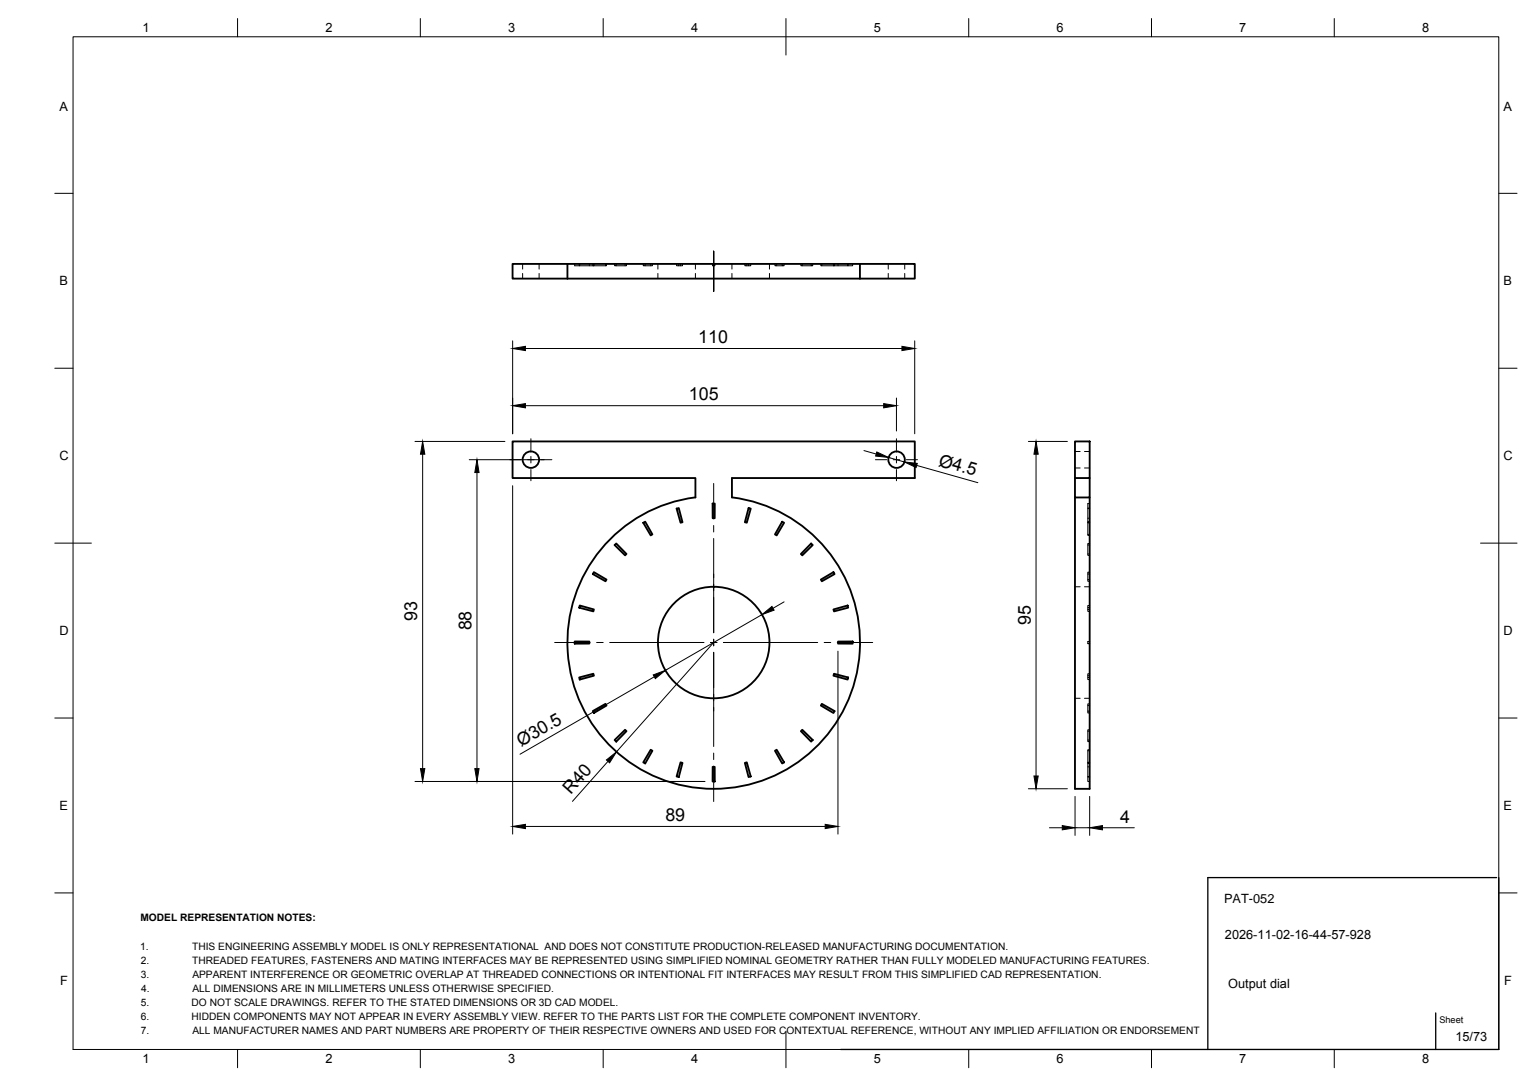
ISO-10303-21;
HEADER;
/* Generated by software containing ST-Developer
 * from STEP Tools, Inc. (www.steptools.com) 
 */

FILE_DESCRIPTION(
/* description */ ('Hand-crank gear train demonstrator'),
/* implementation_level */ '2;1');

FILE_NAME(
/* name */ 'Output dial.step',
/* time_stamp */ '2026-10-28T03:22:13-07:00',
/* author */ (''),
/* organization */ (''),
/* preprocessor_version */ 'ST-DEVELOPER v20.2',
/* originating_system */ 'Autodesk Translation Framework v15.17.0.0',
/* authorisation */ '');

FILE_SCHEMA (('AUTOMOTIVE_DESIGN { 1 0 10303 214 3 1 1 }'));
ENDSEC;

DATA;
#10=MECHANICAL_DESIGN_GEOMETRIC_PRESENTATION_REPRESENTATION('',(#1226),#62758);
#1083=SHAPE_REPRESENTATION_RELATIONSHIP('SRR','None',#63057,#1147);
#1147=ADVANCED_BREP_SHAPE_REPRESENTATION('',(#1303),#62711);
#1226=STYLED_ITEM('',(#63476),#1303);
#1303=MANIFOLD_SOLID_BREP('Body1',#16408);
#1506=FACE_BOUND('',#3606,.T.);
#1507=FACE_BOUND('',#3607,.T.);
#1508=FACE_BOUND('',#3608,.T.);
#1509=FACE_BOUND('',#3611,.T.);
#1510=FACE_BOUND('',#3612,.T.);
#1511=FACE_BOUND('',#3613,.T.);
#1512=FACE_BOUND('',#3614,.T.);
#1513=FACE_BOUND('',#3615,.T.);
#1514=FACE_BOUND('',#3616,.T.);
#1515=FACE_BOUND('',#3617,.T.);
#1516=FACE_BOUND('',#3618,.T.);
#1517=FACE_BOUND('',#3619,.T.);
#1518=FACE_BOUND('',#3620,.T.);
#1519=FACE_BOUND('',#3621,.T.);
#1520=FACE_BOUND('',#3622,.T.);
#1521=FACE_BOUND('',#3623,.T.);
#1522=FACE_BOUND('',#3624,.T.);
#1523=FACE_BOUND('',#3625,.T.);
#1524=FACE_BOUND('',#3626,.T.);
#1525=FACE_BOUND('',#3627,.T.);
#1526=FACE_BOUND('',#3628,.T.);
#1527=FACE_BOUND('',#3629,.T.);
#1528=FACE_BOUND('',#3630,.T.);
#1529=FACE_BOUND('',#3631,.T.);
#1530=FACE_BOUND('',#3632,.T.);
#1531=FACE_BOUND('',#3633,.T.);
#1532=FACE_BOUND('',#3634,.T.);
#1533=FACE_BOUND('',#3635,.T.);
#1534=FACE_BOUND('',#3636,.T.);
#1535=FACE_BOUND('',#3637,.T.);
#1726=PLANE('',#17771);
#1727=PLANE('',#17772);
#1728=PLANE('',#17773);
#1729=PLANE('',#17774);
#1730=PLANE('',#17775);
#1731=PLANE('',#17776);
#1732=PLANE('',#17777);
#1733=PLANE('',#17778);
#1734=PLANE('',#17779);
#1735=PLANE('',#17780);
#1736=PLANE('',#17781);
#1737=PLANE('',#17782);
#1738=PLANE('',#17783);
#1739=PLANE('',#17784);
#1740=PLANE('',#17785);
#1741=PLANE('',#17786);
#1742=PLANE('',#17787);
#1743=PLANE('',#17788);
#1744=PLANE('',#17789);
#1745=PLANE('',#17790);
#1746=PLANE('',#17791);
#1747=PLANE('',#17792);
#1748=PLANE('',#17793);
#1749=PLANE('',#17794);
#1750=PLANE('',#17795);
#1751=PLANE('',#17796);
#1752=PLANE('',#17797);
#1753=PLANE('',#17798);
#1754=PLANE('',#17799);
#1755=PLANE('',#17800);
#1756=PLANE('',#17801);
#1757=PLANE('',#17802);
#1758=PLANE('',#17803);
#1759=PLANE('',#17804);
#1760=PLANE('',#17805);
#1761=PLANE('',#17806);
#1762=PLANE('',#17807);
#1763=PLANE('',#17808);
#1764=PLANE('',#17809);
#1765=PLANE('',#17810);
#1766=PLANE('',#17811);
#1767=PLANE('',#17812);
#1768=PLANE('',#17813);
#1769=PLANE('',#17814);
#1770=PLANE('',#17815);
#1771=PLANE('',#17816);
#1772=PLANE('',#17817);
#1773=PLANE('',#17818);
#1774=PLANE('',#17819);
#1775=PLANE('',#17820);
#1776=PLANE('',#17821);
#1777=PLANE('',#17822);
#1778=PLANE('',#17823);
#1779=PLANE('',#17824);
#1780=PLANE('',#17825);
#1781=PLANE('',#17826);
#1782=PLANE('',#17827);
#1783=PLANE('',#17828);
#1784=PLANE('',#17829);
#1785=PLANE('',#17830);
#1786=PLANE('',#17831);
#1787=PLANE('',#17832);
#1788=PLANE('',#17833);
#1789=PLANE('',#17834);
#1790=PLANE('',#17835);
#1791=PLANE('',#17836);
#1792=PLANE('',#17837);
#1793=PLANE('',#17838);
#1794=PLANE('',#17839);
#1795=PLANE('',#17840);
#1796=PLANE('',#17841);
#1797=PLANE('',#17842);
#1798=PLANE('',#17843);
#1799=PLANE('',#17844);
#1800=PLANE('',#17845);
#1801=PLANE('',#17846);
#1802=PLANE('',#17847);
#1803=PLANE('',#17848);
#1804=PLANE('',#17849);
#1805=PLANE('',#17850);
#1806=PLANE('',#17851);
#1807=PLANE('',#17852);
#1808=PLANE('',#17853);
#1809=PLANE('',#17854);
#1810=PLANE('',#17855);
#1811=PLANE('',#17856);
#1812=PLANE('',#17857);
#1813=PLANE('',#17858);
#1814=PLANE('',#17859);
#1815=PLANE('',#17860);
#1816=PLANE('',#17861);
#1817=PLANE('',#17862);
#1818=PLANE('',#17863);
#1819=PLANE('',#17864);
#1820=PLANE('',#17865);
#1821=PLANE('',#17866);
#1822=PLANE('',#17867);
#1823=PLANE('',#17868);
#1824=PLANE('',#17869);
#1825=PLANE('',#17870);
#1826=PLANE('',#17871);
#1827=PLANE('',#17872);
#1828=PLANE('',#17873);
#1829=PLANE('',#17874);
#1830=PLANE('',#17875);
#1831=PLANE('',#17876);
#1832=PLANE('',#17877);
#1833=PLANE('',#17878);
#1834=PLANE('',#17879);
#1835=PLANE('',#17880);
#1836=PLANE('',#17881);
#1837=PLANE('',#17882);
#1838=PLANE('',#17883);
#1839=PLANE('',#17884);
#1840=PLANE('',#17885);
#1841=PLANE('',#17886);
#1842=PLANE('',#17887);
#1843=PLANE('',#17888);
#1844=PLANE('',#17889);
#1845=PLANE('',#17890);
#1846=PLANE('',#17900);
#1847=PLANE('',#17901);
#1848=PLANE('',#17902);
#1849=PLANE('',#17903);
#1850=PLANE('',#17904);
#1851=PLANE('',#17905);
#1852=PLANE('',#17906);
#1853=PLANE('',#17908);
#1854=PLANE('',#17909);
#2376=FACE_OUTER_BOUND('',#3476,.T.);
#2377=FACE_OUTER_BOUND('',#3477,.T.);
#2378=FACE_OUTER_BOUND('',#3478,.T.);
#2379=FACE_OUTER_BOUND('',#3479,.T.);
#2380=FACE_OUTER_BOUND('',#3480,.T.);
#2381=FACE_OUTER_BOUND('',#3481,.T.);
#2382=FACE_OUTER_BOUND('',#3482,.T.);
#2383=FACE_OUTER_BOUND('',#3483,.T.);
#2384=FACE_OUTER_BOUND('',#3484,.T.);
#2385=FACE_OUTER_BOUND('',#3485,.T.);
#2386=FACE_OUTER_BOUND('',#3486,.T.);
#2387=FACE_OUTER_BOUND('',#3487,.T.);
#2388=FACE_OUTER_BOUND('',#3488,.T.);
#2389=FACE_OUTER_BOUND('',#3489,.T.);
#2390=FACE_OUTER_BOUND('',#3490,.T.);
#2391=FACE_OUTER_BOUND('',#3491,.T.);
#2392=FACE_OUTER_BOUND('',#3492,.T.);
#2393=FACE_OUTER_BOUND('',#3493,.T.);
#2394=FACE_OUTER_BOUND('',#3494,.T.);
#2395=FACE_OUTER_BOUND('',#3495,.T.);
#2396=FACE_OUTER_BOUND('',#3496,.T.);
#2397=FACE_OUTER_BOUND('',#3497,.T.);
#2398=FACE_OUTER_BOUND('',#3498,.T.);
#2399=FACE_OUTER_BOUND('',#3499,.T.);
#2400=FACE_OUTER_BOUND('',#3500,.T.);
#2401=FACE_OUTER_BOUND('',#3501,.T.);
#2402=FACE_OUTER_BOUND('',#3502,.T.);
#2403=FACE_OUTER_BOUND('',#3503,.T.);
#2404=FACE_OUTER_BOUND('',#3504,.T.);
#2405=FACE_OUTER_BOUND('',#3505,.T.);
#2406=FACE_OUTER_BOUND('',#3506,.T.);
#2407=FACE_OUTER_BOUND('',#3507,.T.);
#2408=FACE_OUTER_BOUND('',#3508,.T.);
#2409=FACE_OUTER_BOUND('',#3509,.T.);
#2410=FACE_OUTER_BOUND('',#3510,.T.);
#2411=FACE_OUTER_BOUND('',#3511,.T.);
#2412=FACE_OUTER_BOUND('',#3512,.T.);
#2413=FACE_OUTER_BOUND('',#3513,.T.);
#2414=FACE_OUTER_BOUND('',#3514,.T.);
#2415=FACE_OUTER_BOUND('',#3515,.T.);
#2416=FACE_OUTER_BOUND('',#3516,.T.);
#2417=FACE_OUTER_BOUND('',#3517,.T.);
#2418=FACE_OUTER_BOUND('',#3518,.T.);
#2419=FACE_OUTER_BOUND('',#3519,.T.);
#2420=FACE_OUTER_BOUND('',#3520,.T.);
#2421=FACE_OUTER_BOUND('',#3521,.T.);
#2422=FACE_OUTER_BOUND('',#3522,.T.);
#2423=FACE_OUTER_BOUND('',#3523,.T.);
#2424=FACE_OUTER_BOUND('',#3524,.T.);
#2425=FACE_OUTER_BOUND('',#3525,.T.);
#2426=FACE_OUTER_BOUND('',#3526,.T.);
#2427=FACE_OUTER_BOUND('',#3527,.T.);
#2428=FACE_OUTER_BOUND('',#3528,.T.);
#2429=FACE_OUTER_BOUND('',#3529,.T.);
#2430=FACE_OUTER_BOUND('',#3530,.T.);
#2431=FACE_OUTER_BOUND('',#3531,.T.);
#2432=FACE_OUTER_BOUND('',#3532,.T.);
#2433=FACE_OUTER_BOUND('',#3533,.T.);
#2434=FACE_OUTER_BOUND('',#3534,.T.);
#2435=FACE_OUTER_BOUND('',#3535,.T.);
#2436=FACE_OUTER_BOUND('',#3536,.T.);
#2437=FACE_OUTER_BOUND('',#3537,.T.);
#2438=FACE_OUTER_BOUND('',#3538,.T.);
#2439=FACE_OUTER_BOUND('',#3539,.T.);
#2440=FACE_OUTER_BOUND('',#3540,.T.);
#2441=FACE_OUTER_BOUND('',#3541,.T.);
#2442=FACE_OUTER_BOUND('',#3542,.T.);
#2443=FACE_OUTER_BOUND('',#3543,.T.);
#2444=FACE_OUTER_BOUND('',#3544,.T.);
#2445=FACE_OUTER_BOUND('',#3545,.T.);
#2446=FACE_OUTER_BOUND('',#3546,.T.);
#2447=FACE_OUTER_BOUND('',#3547,.T.);
#2448=FACE_OUTER_BOUND('',#3548,.T.);
#2449=FACE_OUTER_BOUND('',#3549,.T.);
#2450=FACE_OUTER_BOUND('',#3550,.T.);
#2451=FACE_OUTER_BOUND('',#3551,.T.);
#2452=FACE_OUTER_BOUND('',#3552,.T.);
#2453=FACE_OUTER_BOUND('',#3553,.T.);
#2454=FACE_OUTER_BOUND('',#3554,.T.);
#2455=FACE_OUTER_BOUND('',#3555,.T.);
#2456=FACE_OUTER_BOUND('',#3556,.T.);
#2457=FACE_OUTER_BOUND('',#3557,.T.);
#2458=FACE_OUTER_BOUND('',#3558,.T.);
#2459=FACE_OUTER_BOUND('',#3559,.T.);
#2460=FACE_OUTER_BOUND('',#3560,.T.);
#2461=FACE_OUTER_BOUND('',#3561,.T.);
#2462=FACE_OUTER_BOUND('',#3562,.T.);
#2463=FACE_OUTER_BOUND('',#3563,.T.);
#2464=FACE_OUTER_BOUND('',#3564,.T.);
#2465=FACE_OUTER_BOUND('',#3565,.T.);
#2466=FACE_OUTER_BOUND('',#3566,.T.);
#2467=FACE_OUTER_BOUND('',#3567,.T.);
#2468=FACE_OUTER_BOUND('',#3568,.T.);
#2469=FACE_OUTER_BOUND('',#3569,.T.);
#2470=FACE_OUTER_BOUND('',#3570,.T.);
#2471=FACE_OUTER_BOUND('',#3571,.T.);
#2472=FACE_OUTER_BOUND('',#3572,.T.);
#2473=FACE_OUTER_BOUND('',#3573,.T.);
#2474=FACE_OUTER_BOUND('',#3574,.T.);
#2475=FACE_OUTER_BOUND('',#3575,.T.);
#2476=FACE_OUTER_BOUND('',#3576,.T.);
#2477=FACE_OUTER_BOUND('',#3577,.T.);
#2478=FACE_OUTER_BOUND('',#3578,.T.);
#2479=FACE_OUTER_BOUND('',#3579,.T.);
#2480=FACE_OUTER_BOUND('',#3580,.T.);
#2481=FACE_OUTER_BOUND('',#3581,.T.);
#2482=FACE_OUTER_BOUND('',#3582,.T.);
#2483=FACE_OUTER_BOUND('',#3583,.T.);
#2484=FACE_OUTER_BOUND('',#3584,.T.);
#2485=FACE_OUTER_BOUND('',#3585,.T.);
#2486=FACE_OUTER_BOUND('',#3586,.T.);
#2487=FACE_OUTER_BOUND('',#3587,.T.);
#2488=FACE_OUTER_BOUND('',#3588,.T.);
#2489=FACE_OUTER_BOUND('',#3589,.T.);
#2490=FACE_OUTER_BOUND('',#3590,.T.);
#2491=FACE_OUTER_BOUND('',#3591,.T.);
#2492=FACE_OUTER_BOUND('',#3592,.T.);
#2493=FACE_OUTER_BOUND('',#3593,.T.);
#2494=FACE_OUTER_BOUND('',#3594,.T.);
#2495=FACE_OUTER_BOUND('',#3595,.T.);
#2496=FACE_OUTER_BOUND('',#3596,.T.);
#2497=FACE_OUTER_BOUND('',#3597,.T.);
#2498=FACE_OUTER_BOUND('',#3598,.T.);
#2499=FACE_OUTER_BOUND('',#3599,.T.);
#2500=FACE_OUTER_BOUND('',#3600,.T.);
#2501=FACE_OUTER_BOUND('',#3601,.T.);
#2502=FACE_OUTER_BOUND('',#3602,.T.);
#2503=FACE_OUTER_BOUND('',#3603,.T.);
#2504=FACE_OUTER_BOUND('',#3604,.T.);
#2505=FACE_OUTER_BOUND('',#3605,.T.);
#2506=FACE_OUTER_BOUND('',#3609,.T.);
#2507=FACE_OUTER_BOUND('',#3610,.T.);
#2508=FACE_OUTER_BOUND('',#3638,.T.);
#3476=EDGE_LOOP('',(#11929,#11930,#11931,#11932));
#3477=EDGE_LOOP('',(#11933,#11934,#11935,#11936));
#3478=EDGE_LOOP('',(#11937,#11938,#11939,#11940));
#3479=EDGE_LOOP('',(#11941,#11942,#11943,#11944));
#3480=EDGE_LOOP('',(#11945,#11946,#11947,#11948));
#3481=EDGE_LOOP('',(#11949,#11950,#11951,#11952));
#3482=EDGE_LOOP('',(#11953,#11954,#11955,#11956));
#3483=EDGE_LOOP('',(#11957,#11958,#11959,#11960));
#3484=EDGE_LOOP('',(#11961,#11962,#11963,#11964));
#3485=EDGE_LOOP('',(#11965,#11966,#11967,#11968));
#3486=EDGE_LOOP('',(#11969,#11970,#11971,#11972));
#3487=EDGE_LOOP('',(#11973,#11974,#11975,#11976));
#3488=EDGE_LOOP('',(#11977,#11978,#11979,#11980));
#3489=EDGE_LOOP('',(#11981,#11982,#11983,#11984));
#3490=EDGE_LOOP('',(#11985,#11986,#11987,#11988));
#3491=EDGE_LOOP('',(#11989,#11990,#11991,#11992));
#3492=EDGE_LOOP('',(#11993,#11994,#11995,#11996));
#3493=EDGE_LOOP('',(#11997,#11998,#11999,#12000));
#3494=EDGE_LOOP('',(#12001,#12002,#12003,#12004));
#3495=EDGE_LOOP('',(#12005,#12006,#12007,#12008));
#3496=EDGE_LOOP('',(#12009,#12010,#12011,#12012));
#3497=EDGE_LOOP('',(#12013,#12014,#12015,#12016));
#3498=EDGE_LOOP('',(#12017,#12018,#12019,#12020));
#3499=EDGE_LOOP('',(#12021,#12022,#12023,#12024));
#3500=EDGE_LOOP('',(#12025,#12026,#12027,#12028));
#3501=EDGE_LOOP('',(#12029,#12030,#12031,#12032));
#3502=EDGE_LOOP('',(#12033,#12034,#12035,#12036));
#3503=EDGE_LOOP('',(#12037,#12038,#12039,#12040));
#3504=EDGE_LOOP('',(#12041,#12042,#12043,#12044));
#3505=EDGE_LOOP('',(#12045,#12046,#12047,#12048));
#3506=EDGE_LOOP('',(#12049,#12050,#12051,#12052));
#3507=EDGE_LOOP('',(#12053,#12054,#12055,#12056));
#3508=EDGE_LOOP('',(#12057,#12058,#12059,#12060));
#3509=EDGE_LOOP('',(#12061,#12062,#12063,#12064));
#3510=EDGE_LOOP('',(#12065,#12066,#12067,#12068));
#3511=EDGE_LOOP('',(#12069,#12070,#12071,#12072));
#3512=EDGE_LOOP('',(#12073,#12074,#12075,#12076));
#3513=EDGE_LOOP('',(#12077,#12078,#12079,#12080));
#3514=EDGE_LOOP('',(#12081,#12082,#12083,#12084));
#3515=EDGE_LOOP('',(#12085,#12086,#12087,#12088));
#3516=EDGE_LOOP('',(#12089,#12090,#12091,#12092));
#3517=EDGE_LOOP('',(#12093,#12094,#12095,#12096));
#3518=EDGE_LOOP('',(#12097,#12098,#12099,#12100));
#3519=EDGE_LOOP('',(#12101,#12102,#12103,#12104));
#3520=EDGE_LOOP('',(#12105,#12106,#12107,#12108));
#3521=EDGE_LOOP('',(#12109,#12110,#12111,#12112));
#3522=EDGE_LOOP('',(#12113,#12114,#12115,#12116));
#3523=EDGE_LOOP('',(#12117,#12118,#12119,#12120));
#3524=EDGE_LOOP('',(#12121,#12122,#12123,#12124));
#3525=EDGE_LOOP('',(#12125,#12126,#12127,#12128));
#3526=EDGE_LOOP('',(#12129,#12130,#12131,#12132));
#3527=EDGE_LOOP('',(#12133,#12134,#12135,#12136));
#3528=EDGE_LOOP('',(#12137,#12138,#12139,#12140));
#3529=EDGE_LOOP('',(#12141,#12142,#12143,#12144));
#3530=EDGE_LOOP('',(#12145,#12146,#12147,#12148));
#3531=EDGE_LOOP('',(#12149,#12150,#12151,#12152));
#3532=EDGE_LOOP('',(#12153,#12154,#12155,#12156));
#3533=EDGE_LOOP('',(#12157,#12158,#12159,#12160));
#3534=EDGE_LOOP('',(#12161,#12162,#12163,#12164));
#3535=EDGE_LOOP('',(#12165,#12166,#12167,#12168));
#3536=EDGE_LOOP('',(#12169,#12170,#12171,#12172));
#3537=EDGE_LOOP('',(#12173,#12174,#12175,#12176));
#3538=EDGE_LOOP('',(#12177,#12178,#12179,#12180));
#3539=EDGE_LOOP('',(#12181,#12182,#12183,#12184));
#3540=EDGE_LOOP('',(#12185,#12186,#12187,#12188));
#3541=EDGE_LOOP('',(#12189,#12190,#12191,#12192));
#3542=EDGE_LOOP('',(#12193,#12194,#12195,#12196));
#3543=EDGE_LOOP('',(#12197,#12198,#12199,#12200));
#3544=EDGE_LOOP('',(#12201,#12202,#12203,#12204));
#3545=EDGE_LOOP('',(#12205,#12206,#12207,#12208));
#3546=EDGE_LOOP('',(#12209,#12210,#12211,#12212));
#3547=EDGE_LOOP('',(#12213,#12214,#12215,#12216));
#3548=EDGE_LOOP('',(#12217,#12218,#12219,#12220));
#3549=EDGE_LOOP('',(#12221,#12222,#12223,#12224));
#3550=EDGE_LOOP('',(#12225,#12226,#12227,#12228));
#3551=EDGE_LOOP('',(#12229,#12230,#12231,#12232));
#3552=EDGE_LOOP('',(#12233,#12234,#12235,#12236));
#3553=EDGE_LOOP('',(#12237,#12238,#12239,#12240));
#3554=EDGE_LOOP('',(#12241,#12242,#12243,#12244));
#3555=EDGE_LOOP('',(#12245,#12246,#12247,#12248));
#3556=EDGE_LOOP('',(#12249,#12250,#12251,#12252));
#3557=EDGE_LOOP('',(#12253,#12254,#12255,#12256));
#3558=EDGE_LOOP('',(#12257,#12258,#12259,#12260));
#3559=EDGE_LOOP('',(#12261,#12262,#12263,#12264));
#3560=EDGE_LOOP('',(#12265,#12266,#12267,#12268));
#3561=EDGE_LOOP('',(#12269,#12270,#12271,#12272));
#3562=EDGE_LOOP('',(#12273,#12274,#12275,#12276));
#3563=EDGE_LOOP('',(#12277,#12278,#12279,#12280));
#3564=EDGE_LOOP('',(#12281,#12282,#12283,#12284));
#3565=EDGE_LOOP('',(#12285,#12286,#12287,#12288));
#3566=EDGE_LOOP('',(#12289,#12290,#12291,#12292));
#3567=EDGE_LOOP('',(#12293,#12294,#12295,#12296));
#3568=EDGE_LOOP('',(#12297,#12298,#12299,#12300));
#3569=EDGE_LOOP('',(#12301,#12302,#12303,#12304));
#3570=EDGE_LOOP('',(#12305,#12306,#12307,#12308));
#3571=EDGE_LOOP('',(#12309,#12310,#12311,#12312));
#3572=EDGE_LOOP('',(#12313,#12314,#12315,#12316));
#3573=EDGE_LOOP('',(#12317,#12318,#12319,#12320));
#3574=EDGE_LOOP('',(#12321,#12322,#12323,#12324));
#3575=EDGE_LOOP('',(#12325,#12326,#12327,#12328));
#3576=EDGE_LOOP('',(#12329,#12330,#12331,#12332));
#3577=EDGE_LOOP('',(#12333,#12334,#12335,#12336));
#3578=EDGE_LOOP('',(#12337,#12338,#12339,#12340));
#3579=EDGE_LOOP('',(#12341,#12342,#12343,#12344));
#3580=EDGE_LOOP('',(#12345,#12346,#12347,#12348));
#3581=EDGE_LOOP('',(#12349,#12350,#12351,#12352));
#3582=EDGE_LOOP('',(#12353,#12354,#12355,#12356));
#3583=EDGE_LOOP('',(#12357,#12358,#12359,#12360));
#3584=EDGE_LOOP('',(#12361,#12362,#12363,#12364));
#3585=EDGE_LOOP('',(#12365,#12366,#12367,#12368));
#3586=EDGE_LOOP('',(#12369,#12370,#12371,#12372));
#3587=EDGE_LOOP('',(#12373,#12374,#12375,#12376));
#3588=EDGE_LOOP('',(#12377,#12378,#12379,#12380));
#3589=EDGE_LOOP('',(#12381,#12382,#12383,#12384));
#3590=EDGE_LOOP('',(#12385,#12386,#12387,#12388));
#3591=EDGE_LOOP('',(#12389,#12390,#12391,#12392));
#3592=EDGE_LOOP('',(#12393,#12394,#12395,#12396));
#3593=EDGE_LOOP('',(#12397,#12398,#12399,#12400));
#3594=EDGE_LOOP('',(#12401,#12402,#12403,#12404));
#3595=EDGE_LOOP('',(#12405,#12406,#12407,#12408));
#3596=EDGE_LOOP('',(#12409,#12410,#12411,#12412));
#3597=EDGE_LOOP('',(#12413,#12414,#12415,#12416));
#3598=EDGE_LOOP('',(#12417,#12418,#12419,#12420));
#3599=EDGE_LOOP('',(#12421,#12422,#12423,#12424));
#3600=EDGE_LOOP('',(#12425,#12426,#12427,#12428));
#3601=EDGE_LOOP('',(#12429,#12430,#12431,#12432));
#3602=EDGE_LOOP('',(#12433,#12434,#12435,#12436));
#3603=EDGE_LOOP('',(#12437,#12438,#12439,#12440));
#3604=EDGE_LOOP('',(#12441,#12442,#12443,#12444));
#3605=EDGE_LOOP('',(#12445,#12446,#12447,#12448,#12449,#12450,#12451,#12452));
#3606=EDGE_LOOP('',(#12453));
#3607=EDGE_LOOP('',(#12454));
#3608=EDGE_LOOP('',(#12455));
#3609=EDGE_LOOP('',(#12456,#12457,#12458,#12459));
#3610=EDGE_LOOP('',(#12460,#12461,#12462,#12463,#12464,#12465,#12466,#12467));
#3611=EDGE_LOOP('',(#12468,#12469,#12470,#12471));
#3612=EDGE_LOOP('',(#12472,#12473,#12474,#12475));
#3613=EDGE_LOOP('',(#12476,#12477,#12478,#12479));
#3614=EDGE_LOOP('',(#12480,#12481,#12482,#12483));
#3615=EDGE_LOOP('',(#12484,#12485,#12486,#12487));
#3616=EDGE_LOOP('',(#12488,#12489,#12490,#12491));
#3617=EDGE_LOOP('',(#12492,#12493,#12494,#12495));
#3618=EDGE_LOOP('',(#12496,#12497,#12498,#12499));
#3619=EDGE_LOOP('',(#12500,#12501,#12502,#12503));
#3620=EDGE_LOOP('',(#12504,#12505,#12506,#12507));
#3621=EDGE_LOOP('',(#12508,#12509,#12510,#12511));
#3622=EDGE_LOOP('',(#12512,#12513,#12514,#12515));
#3623=EDGE_LOOP('',(#12516,#12517,#12518,#12519));
#3624=EDGE_LOOP('',(#12520,#12521,#12522,#12523));
#3625=EDGE_LOOP('',(#12524));
#3626=EDGE_LOOP('',(#12525));
#3627=EDGE_LOOP('',(#12526));
#3628=EDGE_LOOP('',(#12527,#12528,#12529,#12530));
#3629=EDGE_LOOP('',(#12531,#12532,#12533,#12534));
#3630=EDGE_LOOP('',(#12535,#12536,#12537,#12538));
#3631=EDGE_LOOP('',(#12539,#12540,#12541,#12542));
#3632=EDGE_LOOP('',(#12543,#12544,#12545,#12546));
#3633=EDGE_LOOP('',(#12547,#12548,#12549,#12550));
#3634=EDGE_LOOP('',(#12551,#12552,#12553,#12554));
#3635=EDGE_LOOP('',(#12555,#12556,#12557,#12558));
#3636=EDGE_LOOP('',(#12559,#12560,#12561,#12562));
#3637=EDGE_LOOP('',(#12563,#12564,#12565,#12566));
#3638=EDGE_LOOP('',(#12567,#12568,#12569,#12570));
#4478=LINE('',#25161,#5610);
#4479=LINE('',#25163,#5611);
#4480=LINE('',#25165,#5612);
#4481=LINE('',#25166,#5613);
#4482=LINE('',#25169,#5614);
#4483=LINE('',#25171,#5615);
#4484=LINE('',#25172,#5616);
#4485=LINE('',#25175,#5617);
#4486=LINE('',#25177,#5618);
#4487=LINE('',#25178,#5619);
#4488=LINE('',#25180,#5620);
#4489=LINE('',#25181,#5621);
#4490=LINE('',#25186,#5622);
#4491=LINE('',#25188,#5623);
#4492=LINE('',#25190,#5624);
#4493=LINE('',#25191,#5625);
#4494=LINE('',#25194,#5626);
#4495=LINE('',#25196,#5627);
#4496=LINE('',#25197,#5628);
#4497=LINE('',#25200,#5629);
#4498=LINE('',#25202,#5630);
#4499=LINE('',#25203,#5631);
#4500=LINE('',#25205,#5632);
#4501=LINE('',#25206,#5633);
#4502=LINE('',#25211,#5634);
#4503=LINE('',#25213,#5635);
#4504=LINE('',#25215,#5636);
#4505=LINE('',#25216,#5637);
#4506=LINE('',#25219,#5638);
#4507=LINE('',#25221,#5639);
#4508=LINE('',#25222,#5640);
#4509=LINE('',#25225,#5641);
#4510=LINE('',#25227,#5642);
#4511=LINE('',#25228,#5643);
#4512=LINE('',#25230,#5644);
#4513=LINE('',#25231,#5645);
#4514=LINE('',#25236,#5646);
#4515=LINE('',#25238,#5647);
#4516=LINE('',#25240,#5648);
#4517=LINE('',#25241,#5649);
#4518=LINE('',#25244,#5650);
#4519=LINE('',#25246,#5651);
#4520=LINE('',#25247,#5652);
#4521=LINE('',#25250,#5653);
#4522=LINE('',#25252,#5654);
#4523=LINE('',#25253,#5655);
#4524=LINE('',#25255,#5656);
#4525=LINE('',#25256,#5657);
#4526=LINE('',#25261,#5658);
#4527=LINE('',#25263,#5659);
#4528=LINE('',#25265,#5660);
#4529=LINE('',#25266,#5661);
#4530=LINE('',#25269,#5662);
#4531=LINE('',#25271,#5663);
#4532=LINE('',#25272,#5664);
#4533=LINE('',#25275,#5665);
#4534=LINE('',#25277,#5666);
#4535=LINE('',#25278,#5667);
#4536=LINE('',#25280,#5668);
#4537=LINE('',#25281,#5669);
#4538=LINE('',#25286,#5670);
#4539=LINE('',#25288,#5671);
#4540=LINE('',#25290,#5672);
#4541=LINE('',#25291,#5673);
#4542=LINE('',#25294,#5674);
#4543=LINE('',#25296,#5675);
#4544=LINE('',#25297,#5676);
#4545=LINE('',#25300,#5677);
#4546=LINE('',#25302,#5678);
#4547=LINE('',#25303,#5679);
#4548=LINE('',#25305,#5680);
#4549=LINE('',#25306,#5681);
#4550=LINE('',#25311,#5682);
#4551=LINE('',#25313,#5683);
#4552=LINE('',#25315,#5684);
#4553=LINE('',#25316,#5685);
#4554=LINE('',#25319,#5686);
#4555=LINE('',#25321,#5687);
#4556=LINE('',#25322,#5688);
#4557=LINE('',#25325,#5689);
#4558=LINE('',#25327,#5690);
#4559=LINE('',#25328,#5691);
#4560=LINE('',#25330,#5692);
#4561=LINE('',#25331,#5693);
#4562=LINE('',#25336,#5694);
#4563=LINE('',#25338,#5695);
#4564=LINE('',#25340,#5696);
#4565=LINE('',#25341,#5697);
#4566=LINE('',#25344,#5698);
#4567=LINE('',#25346,#5699);
#4568=LINE('',#25347,#5700);
#4569=LINE('',#25350,#5701);
#4570=LINE('',#25352,#5702);
#4571=LINE('',#25353,#5703);
#4572=LINE('',#25355,#5704);
#4573=LINE('',#25356,#5705);
#4574=LINE('',#25361,#5706);
#4575=LINE('',#25363,#5707);
#4576=LINE('',#25365,#5708);
#4577=LINE('',#25366,#5709);
#4578=LINE('',#25369,#5710);
#4579=LINE('',#25371,#5711);
#4580=LINE('',#25372,#5712);
#4581=LINE('',#25375,#5713);
#4582=LINE('',#25377,#5714);
#4583=LINE('',#25378,#5715);
#4584=LINE('',#25380,#5716);
#4585=LINE('',#25381,#5717);
#4586=LINE('',#25386,#5718);
#4587=LINE('',#25388,#5719);
#4588=LINE('',#25390,#5720);
#4589=LINE('',#25391,#5721);
#4590=LINE('',#25394,#5722);
#4591=LINE('',#25396,#5723);
#4592=LINE('',#25397,#5724);
#4593=LINE('',#25400,#5725);
#4594=LINE('',#25402,#5726);
#4595=LINE('',#25403,#5727);
#4596=LINE('',#25405,#5728);
#4597=LINE('',#25406,#5729);
#4598=LINE('',#25411,#5730);
#4599=LINE('',#25413,#5731);
#4600=LINE('',#25415,#5732);
#4601=LINE('',#25416,#5733);
#4602=LINE('',#25419,#5734);
#4603=LINE('',#25421,#5735);
#4604=LINE('',#25422,#5736);
#4605=LINE('',#25425,#5737);
#4606=LINE('',#25427,#5738);
#4607=LINE('',#25428,#5739);
#4608=LINE('',#25430,#5740);
#4609=LINE('',#25431,#5741);
#4610=LINE('',#25436,#5742);
#4611=LINE('',#25438,#5743);
#4612=LINE('',#25440,#5744);
#4613=LINE('',#25441,#5745);
#4614=LINE('',#25444,#5746);
#4615=LINE('',#25446,#5747);
#4616=LINE('',#25447,#5748);
#4617=LINE('',#25450,#5749);
#4618=LINE('',#25452,#5750);
#4619=LINE('',#25453,#5751);
#4620=LINE('',#25455,#5752);
#4621=LINE('',#25456,#5753);
#4622=LINE('',#25461,#5754);
#4623=LINE('',#25463,#5755);
#4624=LINE('',#25465,#5756);
#4625=LINE('',#25466,#5757);
#4626=LINE('',#25469,#5758);
#4627=LINE('',#25471,#5759);
#4628=LINE('',#25472,#5760);
#4629=LINE('',#25475,#5761);
#4630=LINE('',#25477,#5762);
#4631=LINE('',#25478,#5763);
#4632=LINE('',#25480,#5764);
#4633=LINE('',#25481,#5765);
#4634=LINE('',#25486,#5766);
#4635=LINE('',#25488,#5767);
#4636=LINE('',#25490,#5768);
#4637=LINE('',#25491,#5769);
#4638=LINE('',#25494,#5770);
#4639=LINE('',#25496,#5771);
#4640=LINE('',#25497,#5772);
#4641=LINE('',#25500,#5773);
#4642=LINE('',#25502,#5774);
#4643=LINE('',#25503,#5775);
#4644=LINE('',#25505,#5776);
#4645=LINE('',#25506,#5777);
#4646=LINE('',#25511,#5778);
#4647=LINE('',#25513,#5779);
#4648=LINE('',#25515,#5780);
#4649=LINE('',#25516,#5781);
#4650=LINE('',#25519,#5782);
#4651=LINE('',#25521,#5783);
#4652=LINE('',#25522,#5784);
#4653=LINE('',#25525,#5785);
#4654=LINE('',#25527,#5786);
#4655=LINE('',#25528,#5787);
#4656=LINE('',#25530,#5788);
#4657=LINE('',#25531,#5789);
#4658=LINE('',#25536,#5790);
#4659=LINE('',#25538,#5791);
#4660=LINE('',#25540,#5792);
#4661=LINE('',#25541,#5793);
#4662=LINE('',#25544,#5794);
#4663=LINE('',#25546,#5795);
#4664=LINE('',#25547,#5796);
#4665=LINE('',#25550,#5797);
#4666=LINE('',#25552,#5798);
#4667=LINE('',#25553,#5799);
#4668=LINE('',#25555,#5800);
#4669=LINE('',#25556,#5801);
#4670=LINE('',#25561,#5802);
#4671=LINE('',#25563,#5803);
#4672=LINE('',#25565,#5804);
#4673=LINE('',#25566,#5805);
#4674=LINE('',#25569,#5806);
#4675=LINE('',#25571,#5807);
#4676=LINE('',#25572,#5808);
#4677=LINE('',#25575,#5809);
#4678=LINE('',#25577,#5810);
#4679=LINE('',#25578,#5811);
#4680=LINE('',#25580,#5812);
#4681=LINE('',#25581,#5813);
#4682=LINE('',#25586,#5814);
#4683=LINE('',#25588,#5815);
#4684=LINE('',#25590,#5816);
#4685=LINE('',#25591,#5817);
#4686=LINE('',#25594,#5818);
#4687=LINE('',#25596,#5819);
#4688=LINE('',#25597,#5820);
#4689=LINE('',#25600,#5821);
#4690=LINE('',#25602,#5822);
#4691=LINE('',#25603,#5823);
#4692=LINE('',#25605,#5824);
#4693=LINE('',#25606,#5825);
#4694=LINE('',#25611,#5826);
#4695=LINE('',#25613,#5827);
#4696=LINE('',#25615,#5828);
#4697=LINE('',#25616,#5829);
#4698=LINE('',#25619,#5830);
#4699=LINE('',#25621,#5831);
#4700=LINE('',#25622,#5832);
#4701=LINE('',#25625,#5833);
#4702=LINE('',#25627,#5834);
#4703=LINE('',#25628,#5835);
#4704=LINE('',#25630,#5836);
#4705=LINE('',#25631,#5837);
#4706=LINE('',#25636,#5838);
#4707=LINE('',#25638,#5839);
#4708=LINE('',#25640,#5840);
#4709=LINE('',#25641,#5841);
#4710=LINE('',#25644,#5842);
#4711=LINE('',#25646,#5843);
#4712=LINE('',#25647,#5844);
#4713=LINE('',#25650,#5845);
#4714=LINE('',#25652,#5846);
#4715=LINE('',#25653,#5847);
#4716=LINE('',#25655,#5848);
#4717=LINE('',#25656,#5849);
#4718=LINE('',#25661,#5850);
#4719=LINE('',#25663,#5851);
#4720=LINE('',#25665,#5852);
#4721=LINE('',#25666,#5853);
#4722=LINE('',#25669,#5854);
#4723=LINE('',#25671,#5855);
#4724=LINE('',#25672,#5856);
#4725=LINE('',#25675,#5857);
#4726=LINE('',#25677,#5858);
#4727=LINE('',#25678,#5859);
#4728=LINE('',#25680,#5860);
#4729=LINE('',#25681,#5861);
#4730=LINE('',#25686,#5862);
#4731=LINE('',#25688,#5863);
#4732=LINE('',#25690,#5864);
#4733=LINE('',#25691,#5865);
#4734=LINE('',#25694,#5866);
#4735=LINE('',#25696,#5867);
#4736=LINE('',#25697,#5868);
#4737=LINE('',#25700,#5869);
#4738=LINE('',#25702,#5870);
#4739=LINE('',#25703,#5871);
#4740=LINE('',#25705,#5872);
#4741=LINE('',#25706,#5873);
#4742=LINE('',#25711,#5874);
#4743=LINE('',#25713,#5875);
#4744=LINE('',#25715,#5876);
#4745=LINE('',#25716,#5877);
#4746=LINE('',#25719,#5878);
#4747=LINE('',#25721,#5879);
#4748=LINE('',#25722,#5880);
#4749=LINE('',#25725,#5881);
#4750=LINE('',#25727,#5882);
#4751=LINE('',#25728,#5883);
#4752=LINE('',#25730,#5884);
#4753=LINE('',#25731,#5885);
#4754=LINE('',#25736,#5886);
#4755=LINE('',#25738,#5887);
#4756=LINE('',#25740,#5888);
#4757=LINE('',#25741,#5889);
#4758=LINE('',#25744,#5890);
#4759=LINE('',#25746,#5891);
#4760=LINE('',#25747,#5892);
#4761=LINE('',#25750,#5893);
#4762=LINE('',#25752,#5894);
#4763=LINE('',#25753,#5895);
#4764=LINE('',#25755,#5896);
#4765=LINE('',#25756,#5897);
#4766=LINE('',#25762,#5898);
#4767=LINE('',#25768,#5899);
#4768=LINE('',#25774,#5900);
#4769=LINE('',#25779,#5901);
#4770=LINE('',#25781,#5902);
#4771=LINE('',#25783,#5903);
#4772=LINE('',#25784,#5904);
#4773=LINE('',#25788,#5905);
#4774=LINE('',#25790,#5906);
#4775=LINE('',#25792,#5907);
#4776=LINE('',#25793,#5908);
#4777=LINE('',#25796,#5909);
#4778=LINE('',#25798,#5910);
#4779=LINE('',#25799,#5911);
#4780=LINE('',#25802,#5912);
#4781=LINE('',#25804,#5913);
#4782=LINE('',#25805,#5914);
#4783=LINE('',#25807,#5915);
#4784=LINE('',#25808,#5916);
#4785=LINE('',#25811,#5917);
#4786=LINE('',#25813,#5918);
#4787=LINE('',#25814,#5919);
#4788=LINE('',#25817,#5920);
#4789=LINE('',#25821,#5921);
#4790=LINE('',#25822,#5922);
#5610=VECTOR('',#20251,1.);
#5611=VECTOR('',#20252,1.);
#5612=VECTOR('',#20253,1.);
#5613=VECTOR('',#20254,1.);
#5614=VECTOR('',#20257,1.);
#5615=VECTOR('',#20258,1.);
#5616=VECTOR('',#20259,1.);
#5617=VECTOR('',#20262,1.);
#5618=VECTOR('',#20263,1.);
#5619=VECTOR('',#20264,1.);
#5620=VECTOR('',#20267,1.);
#5621=VECTOR('',#20268,1.);
#5622=VECTOR('',#20273,1.);
#5623=VECTOR('',#20274,1.);
#5624=VECTOR('',#20275,1.);
#5625=VECTOR('',#20276,1.);
#5626=VECTOR('',#20279,1.);
#5627=VECTOR('',#20280,1.);
#5628=VECTOR('',#20281,1.);
#5629=VECTOR('',#20284,1.);
#5630=VECTOR('',#20285,1.);
#5631=VECTOR('',#20286,1.);
#5632=VECTOR('',#20289,1.);
#5633=VECTOR('',#20290,1.);
#5634=VECTOR('',#20295,1.);
#5635=VECTOR('',#20296,1.);
#5636=VECTOR('',#20297,1.);
#5637=VECTOR('',#20298,1.);
#5638=VECTOR('',#20301,1.);
#5639=VECTOR('',#20302,1.);
#5640=VECTOR('',#20303,1.);
#5641=VECTOR('',#20306,1.);
#5642=VECTOR('',#20307,1.);
#5643=VECTOR('',#20308,1.);
#5644=VECTOR('',#20311,1.);
#5645=VECTOR('',#20312,1.);
#5646=VECTOR('',#20317,1.);
#5647=VECTOR('',#20318,1.);
#5648=VECTOR('',#20319,1.);
#5649=VECTOR('',#20320,1.);
#5650=VECTOR('',#20323,1.);
#5651=VECTOR('',#20324,1.);
#5652=VECTOR('',#20325,1.);
#5653=VECTOR('',#20328,1.);
#5654=VECTOR('',#20329,1.);
#5655=VECTOR('',#20330,1.);
#5656=VECTOR('',#20333,1.);
#5657=VECTOR('',#20334,1.);
#5658=VECTOR('',#20339,1.);
#5659=VECTOR('',#20340,1.);
#5660=VECTOR('',#20341,1.);
#5661=VECTOR('',#20342,1.);
#5662=VECTOR('',#20345,1.);
#5663=VECTOR('',#20346,1.);
#5664=VECTOR('',#20347,1.);
#5665=VECTOR('',#20350,1.);
#5666=VECTOR('',#20351,1.);
#5667=VECTOR('',#20352,1.);
#5668=VECTOR('',#20355,1.);
#5669=VECTOR('',#20356,1.);
#5670=VECTOR('',#20361,1.);
#5671=VECTOR('',#20362,1.);
#5672=VECTOR('',#20363,1.);
#5673=VECTOR('',#20364,1.);
#5674=VECTOR('',#20367,1.);
#5675=VECTOR('',#20368,1.);
#5676=VECTOR('',#20369,1.);
#5677=VECTOR('',#20372,1.);
#5678=VECTOR('',#20373,1.);
#5679=VECTOR('',#20374,1.);
#5680=VECTOR('',#20377,1.);
#5681=VECTOR('',#20378,1.);
#5682=VECTOR('',#20383,1.);
#5683=VECTOR('',#20384,1.);
#5684=VECTOR('',#20385,1.);
#5685=VECTOR('',#20386,1.);
#5686=VECTOR('',#20389,1.);
#5687=VECTOR('',#20390,1.);
#5688=VECTOR('',#20391,1.);
#5689=VECTOR('',#20394,1.);
#5690=VECTOR('',#20395,1.);
#5691=VECTOR('',#20396,1.);
#5692=VECTOR('',#20399,1.);
#5693=VECTOR('',#20400,1.);
#5694=VECTOR('',#20405,1.);
#5695=VECTOR('',#20406,1.);
#5696=VECTOR('',#20407,1.);
#5697=VECTOR('',#20408,1.);
#5698=VECTOR('',#20411,1.);
#5699=VECTOR('',#20412,1.);
#5700=VECTOR('',#20413,1.);
#5701=VECTOR('',#20416,1.);
#5702=VECTOR('',#20417,1.);
#5703=VECTOR('',#20418,1.);
#5704=VECTOR('',#20421,1.);
#5705=VECTOR('',#20422,1.);
#5706=VECTOR('',#20427,1.);
#5707=VECTOR('',#20428,1.);
#5708=VECTOR('',#20429,1.);
#5709=VECTOR('',#20430,1.);
#5710=VECTOR('',#20433,1.);
#5711=VECTOR('',#20434,1.);
#5712=VECTOR('',#20435,1.);
#5713=VECTOR('',#20438,1.);
#5714=VECTOR('',#20439,1.);
#5715=VECTOR('',#20440,1.);
#5716=VECTOR('',#20443,1.);
#5717=VECTOR('',#20444,1.);
#5718=VECTOR('',#20449,1.);
#5719=VECTOR('',#20450,1.);
#5720=VECTOR('',#20451,1.);
#5721=VECTOR('',#20452,1.);
#5722=VECTOR('',#20455,1.);
#5723=VECTOR('',#20456,1.);
#5724=VECTOR('',#20457,1.);
#5725=VECTOR('',#20460,1.);
#5726=VECTOR('',#20461,1.);
#5727=VECTOR('',#20462,1.);
#5728=VECTOR('',#20465,1.);
#5729=VECTOR('',#20466,1.);
#5730=VECTOR('',#20471,1.);
#5731=VECTOR('',#20472,1.);
#5732=VECTOR('',#20473,1.);
#5733=VECTOR('',#20474,1.);
#5734=VECTOR('',#20477,1.);
#5735=VECTOR('',#20478,1.);
#5736=VECTOR('',#20479,1.);
#5737=VECTOR('',#20482,1.);
#5738=VECTOR('',#20483,1.);
#5739=VECTOR('',#20484,1.);
#5740=VECTOR('',#20487,1.);
#5741=VECTOR('',#20488,1.);
#5742=VECTOR('',#20493,1.);
#5743=VECTOR('',#20494,1.);
#5744=VECTOR('',#20495,1.);
#5745=VECTOR('',#20496,1.);
#5746=VECTOR('',#20499,1.);
#5747=VECTOR('',#20500,1.);
#5748=VECTOR('',#20501,1.);
#5749=VECTOR('',#20504,1.);
#5750=VECTOR('',#20505,1.);
#5751=VECTOR('',#20506,1.);
#5752=VECTOR('',#20509,1.);
#5753=VECTOR('',#20510,1.);
#5754=VECTOR('',#20515,1.);
#5755=VECTOR('',#20516,1.);
#5756=VECTOR('',#20517,1.);
#5757=VECTOR('',#20518,1.);
#5758=VECTOR('',#20521,1.);
#5759=VECTOR('',#20522,1.);
#5760=VECTOR('',#20523,1.);
#5761=VECTOR('',#20526,1.);
#5762=VECTOR('',#20527,1.);
#5763=VECTOR('',#20528,1.);
#5764=VECTOR('',#20531,1.);
#5765=VECTOR('',#20532,1.);
#5766=VECTOR('',#20537,1.);
#5767=VECTOR('',#20538,1.);
#5768=VECTOR('',#20539,1.);
#5769=VECTOR('',#20540,1.);
#5770=VECTOR('',#20543,1.);
#5771=VECTOR('',#20544,1.);
#5772=VECTOR('',#20545,1.);
#5773=VECTOR('',#20548,1.);
#5774=VECTOR('',#20549,1.);
#5775=VECTOR('',#20550,1.);
#5776=VECTOR('',#20553,1.);
#5777=VECTOR('',#20554,1.);
#5778=VECTOR('',#20559,1.);
#5779=VECTOR('',#20560,1.);
#5780=VECTOR('',#20561,1.);
#5781=VECTOR('',#20562,1.);
#5782=VECTOR('',#20565,1.);
#5783=VECTOR('',#20566,1.);
#5784=VECTOR('',#20567,1.);
#5785=VECTOR('',#20570,1.);
#5786=VECTOR('',#20571,1.);
#5787=VECTOR('',#20572,1.);
#5788=VECTOR('',#20575,1.);
#5789=VECTOR('',#20576,1.);
#5790=VECTOR('',#20581,1.);
#5791=VECTOR('',#20582,1.);
#5792=VECTOR('',#20583,1.);
#5793=VECTOR('',#20584,1.);
#5794=VECTOR('',#20587,1.);
#5795=VECTOR('',#20588,1.);
#5796=VECTOR('',#20589,1.);
#5797=VECTOR('',#20592,1.);
#5798=VECTOR('',#20593,1.);
#5799=VECTOR('',#20594,1.);
#5800=VECTOR('',#20597,1.);
#5801=VECTOR('',#20598,1.);
#5802=VECTOR('',#20603,1.);
#5803=VECTOR('',#20604,1.);
#5804=VECTOR('',#20605,1.);
#5805=VECTOR('',#20606,1.);
#5806=VECTOR('',#20609,1.);
#5807=VECTOR('',#20610,1.);
#5808=VECTOR('',#20611,1.);
#5809=VECTOR('',#20614,1.);
#5810=VECTOR('',#20615,1.);
#5811=VECTOR('',#20616,1.);
#5812=VECTOR('',#20619,1.);
#5813=VECTOR('',#20620,1.);
#5814=VECTOR('',#20625,1.);
#5815=VECTOR('',#20626,1.);
#5816=VECTOR('',#20627,1.);
#5817=VECTOR('',#20628,1.);
#5818=VECTOR('',#20631,1.);
#5819=VECTOR('',#20632,1.);
#5820=VECTOR('',#20633,1.);
#5821=VECTOR('',#20636,1.);
#5822=VECTOR('',#20637,1.);
#5823=VECTOR('',#20638,1.);
#5824=VECTOR('',#20641,1.);
#5825=VECTOR('',#20642,1.);
#5826=VECTOR('',#20647,1.);
#5827=VECTOR('',#20648,1.);
#5828=VECTOR('',#20649,1.);
#5829=VECTOR('',#20650,1.);
#5830=VECTOR('',#20653,1.);
#5831=VECTOR('',#20654,1.);
#5832=VECTOR('',#20655,1.);
#5833=VECTOR('',#20658,1.);
#5834=VECTOR('',#20659,1.);
#5835=VECTOR('',#20660,1.);
#5836=VECTOR('',#20663,1.);
#5837=VECTOR('',#20664,1.);
#5838=VECTOR('',#20669,1.);
#5839=VECTOR('',#20670,1.);
#5840=VECTOR('',#20671,1.);
#5841=VECTOR('',#20672,1.);
#5842=VECTOR('',#20675,1.);
#5843=VECTOR('',#20676,1.);
#5844=VECTOR('',#20677,1.);
#5845=VECTOR('',#20680,1.);
#5846=VECTOR('',#20681,1.);
#5847=VECTOR('',#20682,1.);
#5848=VECTOR('',#20685,1.);
#5849=VECTOR('',#20686,1.);
#5850=VECTOR('',#20691,1.);
#5851=VECTOR('',#20692,1.);
#5852=VECTOR('',#20693,1.);
#5853=VECTOR('',#20694,1.);
#5854=VECTOR('',#20697,1.);
#5855=VECTOR('',#20698,1.);
#5856=VECTOR('',#20699,1.);
#5857=VECTOR('',#20702,1.);
#5858=VECTOR('',#20703,1.);
#5859=VECTOR('',#20704,1.);
#5860=VECTOR('',#20707,1.);
#5861=VECTOR('',#20708,1.);
#5862=VECTOR('',#20713,1.);
#5863=VECTOR('',#20714,1.);
#5864=VECTOR('',#20715,1.);
#5865=VECTOR('',#20716,1.);
#5866=VECTOR('',#20719,1.);
#5867=VECTOR('',#20720,1.);
#5868=VECTOR('',#20721,1.);
#5869=VECTOR('',#20724,1.);
#5870=VECTOR('',#20725,1.);
#5871=VECTOR('',#20726,1.);
#5872=VECTOR('',#20729,1.);
#5873=VECTOR('',#20730,1.);
#5874=VECTOR('',#20735,1.);
#5875=VECTOR('',#20736,1.);
#5876=VECTOR('',#20737,1.);
#5877=VECTOR('',#20738,1.);
#5878=VECTOR('',#20741,1.);
#5879=VECTOR('',#20742,1.);
#5880=VECTOR('',#20743,1.);
#5881=VECTOR('',#20746,1.);
#5882=VECTOR('',#20747,1.);
#5883=VECTOR('',#20748,1.);
#5884=VECTOR('',#20751,1.);
#5885=VECTOR('',#20752,1.);
#5886=VECTOR('',#20757,1.);
#5887=VECTOR('',#20758,1.);
#5888=VECTOR('',#20759,1.);
#5889=VECTOR('',#20760,1.);
#5890=VECTOR('',#20763,1.);
#5891=VECTOR('',#20764,1.);
#5892=VECTOR('',#20765,1.);
#5893=VECTOR('',#20768,1.);
#5894=VECTOR('',#20769,1.);
#5895=VECTOR('',#20770,1.);
#5896=VECTOR('',#20773,1.);
#5897=VECTOR('',#20774,1.);
#5898=VECTOR('',#20781,0.225000000000001);
#5899=VECTOR('',#20788,0.225000000000001);
#5900=VECTOR('',#20795,1.525);
#5901=VECTOR('',#20800,1.);
#5902=VECTOR('',#20801,1.);
#5903=VECTOR('',#20802,1.);
#5904=VECTOR('',#20803,1.);
#5905=VECTOR('',#20806,1.);
#5906=VECTOR('',#20807,1.);
#5907=VECTOR('',#20808,1.);
#5908=VECTOR('',#20809,1.);
#5909=VECTOR('',#20812,1.);
#5910=VECTOR('',#20813,1.);
#5911=VECTOR('',#20814,1.);
#5912=VECTOR('',#20817,1.);
#5913=VECTOR('',#20818,1.);
#5914=VECTOR('',#20819,1.);
#5915=VECTOR('',#20822,1.);
#5916=VECTOR('',#20823,1.);
#5917=VECTOR('',#20826,1.);
#5918=VECTOR('',#20827,1.);
#5919=VECTOR('',#20828,1.);
#5920=VECTOR('',#20831,1.);
#5921=VECTOR('',#20836,1.);
#5922=VECTOR('',#20837,1.);
#6873=CIRCLE('',#17892,0.225000000000001);
#6874=CIRCLE('',#17893,0.225000000000001);
#6875=CIRCLE('',#17895,0.225000000000001);
#6876=CIRCLE('',#17896,0.225000000000001);
#6877=CIRCLE('',#17898,1.525);
#6878=CIRCLE('',#17899,1.525);
#6879=CIRCLE('',#17907,4.);
#6880=CIRCLE('',#17910,4.);
#7592=VERTEX_POINT('',#25159);
#7593=VERTEX_POINT('',#25160);
#7594=VERTEX_POINT('',#25162);
#7595=VERTEX_POINT('',#25164);
#7596=VERTEX_POINT('',#25168);
#7597=VERTEX_POINT('',#25170);
#7598=VERTEX_POINT('',#25174);
#7599=VERTEX_POINT('',#25176);
#7600=VERTEX_POINT('',#25184);
#7601=VERTEX_POINT('',#25185);
#7602=VERTEX_POINT('',#25187);
#7603=VERTEX_POINT('',#25189);
#7604=VERTEX_POINT('',#25193);
#7605=VERTEX_POINT('',#25195);
#7606=VERTEX_POINT('',#25199);
#7607=VERTEX_POINT('',#25201);
#7608=VERTEX_POINT('',#25209);
#7609=VERTEX_POINT('',#25210);
#7610=VERTEX_POINT('',#25212);
#7611=VERTEX_POINT('',#25214);
#7612=VERTEX_POINT('',#25218);
#7613=VERTEX_POINT('',#25220);
#7614=VERTEX_POINT('',#25224);
#7615=VERTEX_POINT('',#25226);
#7616=VERTEX_POINT('',#25234);
#7617=VERTEX_POINT('',#25235);
#7618=VERTEX_POINT('',#25237);
#7619=VERTEX_POINT('',#25239);
#7620=VERTEX_POINT('',#25243);
#7621=VERTEX_POINT('',#25245);
#7622=VERTEX_POINT('',#25249);
#7623=VERTEX_POINT('',#25251);
#7624=VERTEX_POINT('',#25259);
#7625=VERTEX_POINT('',#25260);
#7626=VERTEX_POINT('',#25262);
#7627=VERTEX_POINT('',#25264);
#7628=VERTEX_POINT('',#25268);
#7629=VERTEX_POINT('',#25270);
#7630=VERTEX_POINT('',#25274);
#7631=VERTEX_POINT('',#25276);
#7632=VERTEX_POINT('',#25284);
#7633=VERTEX_POINT('',#25285);
#7634=VERTEX_POINT('',#25287);
#7635=VERTEX_POINT('',#25289);
#7636=VERTEX_POINT('',#25293);
#7637=VERTEX_POINT('',#25295);
#7638=VERTEX_POINT('',#25299);
#7639=VERTEX_POINT('',#25301);
#7640=VERTEX_POINT('',#25309);
#7641=VERTEX_POINT('',#25310);
#7642=VERTEX_POINT('',#25312);
#7643=VERTEX_POINT('',#25314);
#7644=VERTEX_POINT('',#25318);
#7645=VERTEX_POINT('',#25320);
#7646=VERTEX_POINT('',#25324);
#7647=VERTEX_POINT('',#25326);
#7648=VERTEX_POINT('',#25334);
#7649=VERTEX_POINT('',#25335);
#7650=VERTEX_POINT('',#25337);
#7651=VERTEX_POINT('',#25339);
#7652=VERTEX_POINT('',#25343);
#7653=VERTEX_POINT('',#25345);
#7654=VERTEX_POINT('',#25349);
#7655=VERTEX_POINT('',#25351);
#7656=VERTEX_POINT('',#25359);
#7657=VERTEX_POINT('',#25360);
#7658=VERTEX_POINT('',#25362);
#7659=VERTEX_POINT('',#25364);
#7660=VERTEX_POINT('',#25368);
#7661=VERTEX_POINT('',#25370);
#7662=VERTEX_POINT('',#25374);
#7663=VERTEX_POINT('',#25376);
#7664=VERTEX_POINT('',#25384);
#7665=VERTEX_POINT('',#25385);
#7666=VERTEX_POINT('',#25387);
#7667=VERTEX_POINT('',#25389);
#7668=VERTEX_POINT('',#25393);
#7669=VERTEX_POINT('',#25395);
#7670=VERTEX_POINT('',#25399);
#7671=VERTEX_POINT('',#25401);
#7672=VERTEX_POINT('',#25409);
#7673=VERTEX_POINT('',#25410);
#7674=VERTEX_POINT('',#25412);
#7675=VERTEX_POINT('',#25414);
#7676=VERTEX_POINT('',#25418);
#7677=VERTEX_POINT('',#25420);
#7678=VERTEX_POINT('',#25424);
#7679=VERTEX_POINT('',#25426);
#7680=VERTEX_POINT('',#25434);
#7681=VERTEX_POINT('',#25435);
#7682=VERTEX_POINT('',#25437);
#7683=VERTEX_POINT('',#25439);
#7684=VERTEX_POINT('',#25443);
#7685=VERTEX_POINT('',#25445);
#7686=VERTEX_POINT('',#25449);
#7687=VERTEX_POINT('',#25451);
#7688=VERTEX_POINT('',#25459);
#7689=VERTEX_POINT('',#25460);
#7690=VERTEX_POINT('',#25462);
#7691=VERTEX_POINT('',#25464);
#7692=VERTEX_POINT('',#25468);
#7693=VERTEX_POINT('',#25470);
#7694=VERTEX_POINT('',#25474);
#7695=VERTEX_POINT('',#25476);
#7696=VERTEX_POINT('',#25484);
#7697=VERTEX_POINT('',#25485);
#7698=VERTEX_POINT('',#25487);
#7699=VERTEX_POINT('',#25489);
#7700=VERTEX_POINT('',#25493);
#7701=VERTEX_POINT('',#25495);
#7702=VERTEX_POINT('',#25499);
#7703=VERTEX_POINT('',#25501);
#7704=VERTEX_POINT('',#25509);
#7705=VERTEX_POINT('',#25510);
#7706=VERTEX_POINT('',#25512);
#7707=VERTEX_POINT('',#25514);
#7708=VERTEX_POINT('',#25518);
#7709=VERTEX_POINT('',#25520);
#7710=VERTEX_POINT('',#25524);
#7711=VERTEX_POINT('',#25526);
#7712=VERTEX_POINT('',#25534);
#7713=VERTEX_POINT('',#25535);
#7714=VERTEX_POINT('',#25537);
#7715=VERTEX_POINT('',#25539);
#7716=VERTEX_POINT('',#25543);
#7717=VERTEX_POINT('',#25545);
#7718=VERTEX_POINT('',#25549);
#7719=VERTEX_POINT('',#25551);
#7720=VERTEX_POINT('',#25559);
#7721=VERTEX_POINT('',#25560);
#7722=VERTEX_POINT('',#25562);
#7723=VERTEX_POINT('',#25564);
#7724=VERTEX_POINT('',#25568);
#7725=VERTEX_POINT('',#25570);
#7726=VERTEX_POINT('',#25574);
#7727=VERTEX_POINT('',#25576);
#7728=VERTEX_POINT('',#25584);
#7729=VERTEX_POINT('',#25585);
#7730=VERTEX_POINT('',#25587);
#7731=VERTEX_POINT('',#25589);
#7732=VERTEX_POINT('',#25593);
#7733=VERTEX_POINT('',#25595);
#7734=VERTEX_POINT('',#25599);
#7735=VERTEX_POINT('',#25601);
#7736=VERTEX_POINT('',#25609);
#7737=VERTEX_POINT('',#25610);
#7738=VERTEX_POINT('',#25612);
#7739=VERTEX_POINT('',#25614);
#7740=VERTEX_POINT('',#25618);
#7741=VERTEX_POINT('',#25620);
#7742=VERTEX_POINT('',#25624);
#7743=VERTEX_POINT('',#25626);
#7744=VERTEX_POINT('',#25634);
#7745=VERTEX_POINT('',#25635);
#7746=VERTEX_POINT('',#25637);
#7747=VERTEX_POINT('',#25639);
#7748=VERTEX_POINT('',#25643);
#7749=VERTEX_POINT('',#25645);
#7750=VERTEX_POINT('',#25649);
#7751=VERTEX_POINT('',#25651);
#7752=VERTEX_POINT('',#25659);
#7753=VERTEX_POINT('',#25660);
#7754=VERTEX_POINT('',#25662);
#7755=VERTEX_POINT('',#25664);
#7756=VERTEX_POINT('',#25668);
#7757=VERTEX_POINT('',#25670);
#7758=VERTEX_POINT('',#25674);
#7759=VERTEX_POINT('',#25676);
#7760=VERTEX_POINT('',#25684);
#7761=VERTEX_POINT('',#25685);
#7762=VERTEX_POINT('',#25687);
#7763=VERTEX_POINT('',#25689);
#7764=VERTEX_POINT('',#25693);
#7765=VERTEX_POINT('',#25695);
#7766=VERTEX_POINT('',#25699);
#7767=VERTEX_POINT('',#25701);
#7768=VERTEX_POINT('',#25709);
#7769=VERTEX_POINT('',#25710);
#7770=VERTEX_POINT('',#25712);
#7771=VERTEX_POINT('',#25714);
#7772=VERTEX_POINT('',#25718);
#7773=VERTEX_POINT('',#25720);
#7774=VERTEX_POINT('',#25724);
#7775=VERTEX_POINT('',#25726);
#7776=VERTEX_POINT('',#25734);
#7777=VERTEX_POINT('',#25735);
#7778=VERTEX_POINT('',#25737);
#7779=VERTEX_POINT('',#25739);
#7780=VERTEX_POINT('',#25743);
#7781=VERTEX_POINT('',#25745);
#7782=VERTEX_POINT('',#25749);
#7783=VERTEX_POINT('',#25751);
#7784=VERTEX_POINT('',#25759);
#7785=VERTEX_POINT('',#25761);
#7786=VERTEX_POINT('',#25765);
#7787=VERTEX_POINT('',#25767);
#7788=VERTEX_POINT('',#25771);
#7789=VERTEX_POINT('',#25773);
#7790=VERTEX_POINT('',#25777);
#7791=VERTEX_POINT('',#25778);
#7792=VERTEX_POINT('',#25780);
#7793=VERTEX_POINT('',#25782);
#7794=VERTEX_POINT('',#25786);
#7795=VERTEX_POINT('',#25787);
#7796=VERTEX_POINT('',#25789);
#7797=VERTEX_POINT('',#25791);
#7798=VERTEX_POINT('',#25795);
#7799=VERTEX_POINT('',#25797);
#7800=VERTEX_POINT('',#25801);
#7801=VERTEX_POINT('',#25803);
#7802=VERTEX_POINT('',#25810);
#7803=VERTEX_POINT('',#25812);
#7804=VERTEX_POINT('',#25816);
#7805=VERTEX_POINT('',#25820);
#9216=EDGE_CURVE('',#7592,#7593,#4478,.T.);
#9217=EDGE_CURVE('',#7594,#7592,#4479,.T.);
#9218=EDGE_CURVE('',#7594,#7595,#4480,.T.);
#9219=EDGE_CURVE('',#7595,#7593,#4481,.T.);
#9220=EDGE_CURVE('',#7593,#7596,#4482,.T.);
#9221=EDGE_CURVE('',#7595,#7597,#4483,.T.);
#9222=EDGE_CURVE('',#7597,#7596,#4484,.T.);
#9223=EDGE_CURVE('',#7596,#7598,#4485,.T.);
#9224=EDGE_CURVE('',#7597,#7599,#4486,.T.);
#9225=EDGE_CURVE('',#7599,#7598,#4487,.T.);
#9226=EDGE_CURVE('',#7598,#7592,#4488,.T.);
#9227=EDGE_CURVE('',#7599,#7594,#4489,.T.);
#9228=EDGE_CURVE('',#7600,#7601,#4490,.T.);
#9229=EDGE_CURVE('',#7602,#7600,#4491,.T.);
#9230=EDGE_CURVE('',#7602,#7603,#4492,.T.);
#9231=EDGE_CURVE('',#7603,#7601,#4493,.T.);
#9232=EDGE_CURVE('',#7601,#7604,#4494,.T.);
#9233=EDGE_CURVE('',#7603,#7605,#4495,.T.);
#9234=EDGE_CURVE('',#7605,#7604,#4496,.T.);
#9235=EDGE_CURVE('',#7604,#7606,#4497,.T.);
#9236=EDGE_CURVE('',#7605,#7607,#4498,.T.);
#9237=EDGE_CURVE('',#7607,#7606,#4499,.T.);
#9238=EDGE_CURVE('',#7606,#7600,#4500,.T.);
#9239=EDGE_CURVE('',#7607,#7602,#4501,.T.);
#9240=EDGE_CURVE('',#7608,#7609,#4502,.T.);
#9241=EDGE_CURVE('',#7610,#7608,#4503,.T.);
#9242=EDGE_CURVE('',#7610,#7611,#4504,.T.);
#9243=EDGE_CURVE('',#7611,#7609,#4505,.T.);
#9244=EDGE_CURVE('',#7609,#7612,#4506,.T.);
#9245=EDGE_CURVE('',#7611,#7613,#4507,.T.);
#9246=EDGE_CURVE('',#7613,#7612,#4508,.T.);
#9247=EDGE_CURVE('',#7612,#7614,#4509,.T.);
#9248=EDGE_CURVE('',#7613,#7615,#4510,.T.);
#9249=EDGE_CURVE('',#7615,#7614,#4511,.T.);
#9250=EDGE_CURVE('',#7614,#7608,#4512,.T.);
#9251=EDGE_CURVE('',#7615,#7610,#4513,.T.);
#9252=EDGE_CURVE('',#7616,#7617,#4514,.T.);
#9253=EDGE_CURVE('',#7618,#7616,#4515,.T.);
#9254=EDGE_CURVE('',#7618,#7619,#4516,.T.);
#9255=EDGE_CURVE('',#7619,#7617,#4517,.T.);
#9256=EDGE_CURVE('',#7617,#7620,#4518,.T.);
#9257=EDGE_CURVE('',#7619,#7621,#4519,.T.);
#9258=EDGE_CURVE('',#7621,#7620,#4520,.T.);
#9259=EDGE_CURVE('',#7620,#7622,#4521,.T.);
#9260=EDGE_CURVE('',#7621,#7623,#4522,.T.);
#9261=EDGE_CURVE('',#7623,#7622,#4523,.T.);
#9262=EDGE_CURVE('',#7622,#7616,#4524,.T.);
#9263=EDGE_CURVE('',#7623,#7618,#4525,.T.);
#9264=EDGE_CURVE('',#7624,#7625,#4526,.T.);
#9265=EDGE_CURVE('',#7626,#7624,#4527,.T.);
#9266=EDGE_CURVE('',#7626,#7627,#4528,.T.);
#9267=EDGE_CURVE('',#7627,#7625,#4529,.T.);
#9268=EDGE_CURVE('',#7625,#7628,#4530,.T.);
#9269=EDGE_CURVE('',#7627,#7629,#4531,.T.);
#9270=EDGE_CURVE('',#7629,#7628,#4532,.T.);
#9271=EDGE_CURVE('',#7628,#7630,#4533,.T.);
#9272=EDGE_CURVE('',#7629,#7631,#4534,.T.);
#9273=EDGE_CURVE('',#7631,#7630,#4535,.T.);
#9274=EDGE_CURVE('',#7630,#7624,#4536,.T.);
#9275=EDGE_CURVE('',#7631,#7626,#4537,.T.);
#9276=EDGE_CURVE('',#7632,#7633,#4538,.T.);
#9277=EDGE_CURVE('',#7634,#7632,#4539,.T.);
#9278=EDGE_CURVE('',#7634,#7635,#4540,.T.);
#9279=EDGE_CURVE('',#7635,#7633,#4541,.T.);
#9280=EDGE_CURVE('',#7633,#7636,#4542,.T.);
#9281=EDGE_CURVE('',#7635,#7637,#4543,.T.);
#9282=EDGE_CURVE('',#7637,#7636,#4544,.T.);
#9283=EDGE_CURVE('',#7636,#7638,#4545,.T.);
#9284=EDGE_CURVE('',#7637,#7639,#4546,.T.);
#9285=EDGE_CURVE('',#7639,#7638,#4547,.T.);
#9286=EDGE_CURVE('',#7638,#7632,#4548,.T.);
#9287=EDGE_CURVE('',#7639,#7634,#4549,.T.);
#9288=EDGE_CURVE('',#7640,#7641,#4550,.T.);
#9289=EDGE_CURVE('',#7642,#7640,#4551,.T.);
#9290=EDGE_CURVE('',#7642,#7643,#4552,.T.);
#9291=EDGE_CURVE('',#7643,#7641,#4553,.T.);
#9292=EDGE_CURVE('',#7641,#7644,#4554,.T.);
#9293=EDGE_CURVE('',#7643,#7645,#4555,.T.);
#9294=EDGE_CURVE('',#7645,#7644,#4556,.T.);
#9295=EDGE_CURVE('',#7644,#7646,#4557,.T.);
#9296=EDGE_CURVE('',#7645,#7647,#4558,.T.);
#9297=EDGE_CURVE('',#7647,#7646,#4559,.T.);
#9298=EDGE_CURVE('',#7646,#7640,#4560,.T.);
#9299=EDGE_CURVE('',#7647,#7642,#4561,.T.);
#9300=EDGE_CURVE('',#7648,#7649,#4562,.T.);
#9301=EDGE_CURVE('',#7650,#7648,#4563,.T.);
#9302=EDGE_CURVE('',#7650,#7651,#4564,.T.);
#9303=EDGE_CURVE('',#7651,#7649,#4565,.T.);
#9304=EDGE_CURVE('',#7649,#7652,#4566,.T.);
#9305=EDGE_CURVE('',#7651,#7653,#4567,.T.);
#9306=EDGE_CURVE('',#7653,#7652,#4568,.T.);
#9307=EDGE_CURVE('',#7652,#7654,#4569,.T.);
#9308=EDGE_CURVE('',#7653,#7655,#4570,.T.);
#9309=EDGE_CURVE('',#7655,#7654,#4571,.T.);
#9310=EDGE_CURVE('',#7654,#7648,#4572,.T.);
#9311=EDGE_CURVE('',#7655,#7650,#4573,.T.);
#9312=EDGE_CURVE('',#7656,#7657,#4574,.T.);
#9313=EDGE_CURVE('',#7658,#7656,#4575,.T.);
#9314=EDGE_CURVE('',#7658,#7659,#4576,.T.);
#9315=EDGE_CURVE('',#7659,#7657,#4577,.T.);
#9316=EDGE_CURVE('',#7657,#7660,#4578,.T.);
#9317=EDGE_CURVE('',#7659,#7661,#4579,.T.);
#9318=EDGE_CURVE('',#7661,#7660,#4580,.T.);
#9319=EDGE_CURVE('',#7660,#7662,#4581,.T.);
#9320=EDGE_CURVE('',#7661,#7663,#4582,.T.);
#9321=EDGE_CURVE('',#7663,#7662,#4583,.T.);
#9322=EDGE_CURVE('',#7662,#7656,#4584,.T.);
#9323=EDGE_CURVE('',#7663,#7658,#4585,.T.);
#9324=EDGE_CURVE('',#7664,#7665,#4586,.T.);
#9325=EDGE_CURVE('',#7666,#7664,#4587,.T.);
#9326=EDGE_CURVE('',#7666,#7667,#4588,.T.);
#9327=EDGE_CURVE('',#7667,#7665,#4589,.T.);
#9328=EDGE_CURVE('',#7665,#7668,#4590,.T.);
#9329=EDGE_CURVE('',#7667,#7669,#4591,.T.);
#9330=EDGE_CURVE('',#7669,#7668,#4592,.T.);
#9331=EDGE_CURVE('',#7668,#7670,#4593,.T.);
#9332=EDGE_CURVE('',#7669,#7671,#4594,.T.);
#9333=EDGE_CURVE('',#7671,#7670,#4595,.T.);
#9334=EDGE_CURVE('',#7670,#7664,#4596,.T.);
#9335=EDGE_CURVE('',#7671,#7666,#4597,.T.);
#9336=EDGE_CURVE('',#7672,#7673,#4598,.T.);
#9337=EDGE_CURVE('',#7674,#7672,#4599,.T.);
#9338=EDGE_CURVE('',#7674,#7675,#4600,.T.);
#9339=EDGE_CURVE('',#7675,#7673,#4601,.T.);
#9340=EDGE_CURVE('',#7673,#7676,#4602,.T.);
#9341=EDGE_CURVE('',#7675,#7677,#4603,.T.);
#9342=EDGE_CURVE('',#7677,#7676,#4604,.T.);
#9343=EDGE_CURVE('',#7676,#7678,#4605,.T.);
#9344=EDGE_CURVE('',#7677,#7679,#4606,.T.);
#9345=EDGE_CURVE('',#7679,#7678,#4607,.T.);
#9346=EDGE_CURVE('',#7678,#7672,#4608,.T.);
#9347=EDGE_CURVE('',#7679,#7674,#4609,.T.);
#9348=EDGE_CURVE('',#7680,#7681,#4610,.T.);
#9349=EDGE_CURVE('',#7682,#7680,#4611,.T.);
#9350=EDGE_CURVE('',#7682,#7683,#4612,.T.);
#9351=EDGE_CURVE('',#7683,#7681,#4613,.T.);
#9352=EDGE_CURVE('',#7681,#7684,#4614,.T.);
#9353=EDGE_CURVE('',#7683,#7685,#4615,.T.);
#9354=EDGE_CURVE('',#7685,#7684,#4616,.T.);
#9355=EDGE_CURVE('',#7684,#7686,#4617,.T.);
#9356=EDGE_CURVE('',#7685,#7687,#4618,.T.);
#9357=EDGE_CURVE('',#7687,#7686,#4619,.T.);
#9358=EDGE_CURVE('',#7686,#7680,#4620,.T.);
#9359=EDGE_CURVE('',#7687,#7682,#4621,.T.);
#9360=EDGE_CURVE('',#7688,#7689,#4622,.T.);
#9361=EDGE_CURVE('',#7690,#7688,#4623,.T.);
#9362=EDGE_CURVE('',#7690,#7691,#4624,.T.);
#9363=EDGE_CURVE('',#7691,#7689,#4625,.T.);
#9364=EDGE_CURVE('',#7689,#7692,#4626,.T.);
#9365=EDGE_CURVE('',#7691,#7693,#4627,.T.);
#9366=EDGE_CURVE('',#7693,#7692,#4628,.T.);
#9367=EDGE_CURVE('',#7692,#7694,#4629,.T.);
#9368=EDGE_CURVE('',#7693,#7695,#4630,.T.);
#9369=EDGE_CURVE('',#7695,#7694,#4631,.T.);
#9370=EDGE_CURVE('',#7694,#7688,#4632,.T.);
#9371=EDGE_CURVE('',#7695,#7690,#4633,.T.);
#9372=EDGE_CURVE('',#7696,#7697,#4634,.T.);
#9373=EDGE_CURVE('',#7698,#7696,#4635,.T.);
#9374=EDGE_CURVE('',#7698,#7699,#4636,.T.);
#9375=EDGE_CURVE('',#7699,#7697,#4637,.T.);
#9376=EDGE_CURVE('',#7697,#7700,#4638,.T.);
#9377=EDGE_CURVE('',#7699,#7701,#4639,.T.);
#9378=EDGE_CURVE('',#7701,#7700,#4640,.T.);
#9379=EDGE_CURVE('',#7700,#7702,#4641,.T.);
#9380=EDGE_CURVE('',#7701,#7703,#4642,.T.);
#9381=EDGE_CURVE('',#7703,#7702,#4643,.T.);
#9382=EDGE_CURVE('',#7702,#7696,#4644,.T.);
#9383=EDGE_CURVE('',#7703,#7698,#4645,.T.);
#9384=EDGE_CURVE('',#7704,#7705,#4646,.T.);
#9385=EDGE_CURVE('',#7706,#7704,#4647,.T.);
#9386=EDGE_CURVE('',#7706,#7707,#4648,.T.);
#9387=EDGE_CURVE('',#7707,#7705,#4649,.T.);
#9388=EDGE_CURVE('',#7705,#7708,#4650,.T.);
#9389=EDGE_CURVE('',#7707,#7709,#4651,.T.);
#9390=EDGE_CURVE('',#7709,#7708,#4652,.T.);
#9391=EDGE_CURVE('',#7708,#7710,#4653,.T.);
#9392=EDGE_CURVE('',#7709,#7711,#4654,.T.);
#9393=EDGE_CURVE('',#7711,#7710,#4655,.T.);
#9394=EDGE_CURVE('',#7710,#7704,#4656,.T.);
#9395=EDGE_CURVE('',#7711,#7706,#4657,.T.);
#9396=EDGE_CURVE('',#7712,#7713,#4658,.T.);
#9397=EDGE_CURVE('',#7714,#7712,#4659,.T.);
#9398=EDGE_CURVE('',#7714,#7715,#4660,.T.);
#9399=EDGE_CURVE('',#7715,#7713,#4661,.T.);
#9400=EDGE_CURVE('',#7713,#7716,#4662,.T.);
#9401=EDGE_CURVE('',#7715,#7717,#4663,.T.);
#9402=EDGE_CURVE('',#7717,#7716,#4664,.T.);
#9403=EDGE_CURVE('',#7716,#7718,#4665,.T.);
#9404=EDGE_CURVE('',#7717,#7719,#4666,.T.);
#9405=EDGE_CURVE('',#7719,#7718,#4667,.T.);
#9406=EDGE_CURVE('',#7718,#7712,#4668,.T.);
#9407=EDGE_CURVE('',#7719,#7714,#4669,.T.);
#9408=EDGE_CURVE('',#7720,#7721,#4670,.T.);
#9409=EDGE_CURVE('',#7722,#7720,#4671,.T.);
#9410=EDGE_CURVE('',#7722,#7723,#4672,.T.);
#9411=EDGE_CURVE('',#7723,#7721,#4673,.T.);
#9412=EDGE_CURVE('',#7721,#7724,#4674,.T.);
#9413=EDGE_CURVE('',#7723,#7725,#4675,.T.);
#9414=EDGE_CURVE('',#7725,#7724,#4676,.T.);
#9415=EDGE_CURVE('',#7724,#7726,#4677,.T.);
#9416=EDGE_CURVE('',#7725,#7727,#4678,.T.);
#9417=EDGE_CURVE('',#7727,#7726,#4679,.T.);
#9418=EDGE_CURVE('',#7726,#7720,#4680,.T.);
#9419=EDGE_CURVE('',#7727,#7722,#4681,.T.);
#9420=EDGE_CURVE('',#7728,#7729,#4682,.T.);
#9421=EDGE_CURVE('',#7730,#7728,#4683,.T.);
#9422=EDGE_CURVE('',#7730,#7731,#4684,.T.);
#9423=EDGE_CURVE('',#7731,#7729,#4685,.T.);
#9424=EDGE_CURVE('',#7729,#7732,#4686,.T.);
#9425=EDGE_CURVE('',#7731,#7733,#4687,.T.);
#9426=EDGE_CURVE('',#7733,#7732,#4688,.T.);
#9427=EDGE_CURVE('',#7732,#7734,#4689,.T.);
#9428=EDGE_CURVE('',#7733,#7735,#4690,.T.);
#9429=EDGE_CURVE('',#7735,#7734,#4691,.T.);
#9430=EDGE_CURVE('',#7734,#7728,#4692,.T.);
#9431=EDGE_CURVE('',#7735,#7730,#4693,.T.);
#9432=EDGE_CURVE('',#7736,#7737,#4694,.T.);
#9433=EDGE_CURVE('',#7738,#7736,#4695,.T.);
#9434=EDGE_CURVE('',#7738,#7739,#4696,.T.);
#9435=EDGE_CURVE('',#7739,#7737,#4697,.T.);
#9436=EDGE_CURVE('',#7737,#7740,#4698,.T.);
#9437=EDGE_CURVE('',#7739,#7741,#4699,.T.);
#9438=EDGE_CURVE('',#7741,#7740,#4700,.T.);
#9439=EDGE_CURVE('',#7740,#7742,#4701,.T.);
#9440=EDGE_CURVE('',#7741,#7743,#4702,.T.);
#9441=EDGE_CURVE('',#7743,#7742,#4703,.T.);
#9442=EDGE_CURVE('',#7742,#7736,#4704,.T.);
#9443=EDGE_CURVE('',#7743,#7738,#4705,.T.);
#9444=EDGE_CURVE('',#7744,#7745,#4706,.T.);
#9445=EDGE_CURVE('',#7746,#7744,#4707,.T.);
#9446=EDGE_CURVE('',#7746,#7747,#4708,.T.);
#9447=EDGE_CURVE('',#7747,#7745,#4709,.T.);
#9448=EDGE_CURVE('',#7745,#7748,#4710,.T.);
#9449=EDGE_CURVE('',#7747,#7749,#4711,.T.);
#9450=EDGE_CURVE('',#7749,#7748,#4712,.T.);
#9451=EDGE_CURVE('',#7748,#7750,#4713,.T.);
#9452=EDGE_CURVE('',#7749,#7751,#4714,.T.);
#9453=EDGE_CURVE('',#7751,#7750,#4715,.T.);
#9454=EDGE_CURVE('',#7750,#7744,#4716,.T.);
#9455=EDGE_CURVE('',#7751,#7746,#4717,.T.);
#9456=EDGE_CURVE('',#7752,#7753,#4718,.T.);
#9457=EDGE_CURVE('',#7754,#7752,#4719,.T.);
#9458=EDGE_CURVE('',#7754,#7755,#4720,.T.);
#9459=EDGE_CURVE('',#7755,#7753,#4721,.T.);
#9460=EDGE_CURVE('',#7753,#7756,#4722,.T.);
#9461=EDGE_CURVE('',#7755,#7757,#4723,.T.);
#9462=EDGE_CURVE('',#7757,#7756,#4724,.T.);
#9463=EDGE_CURVE('',#7756,#7758,#4725,.T.);
#9464=EDGE_CURVE('',#7757,#7759,#4726,.T.);
#9465=EDGE_CURVE('',#7759,#7758,#4727,.T.);
#9466=EDGE_CURVE('',#7758,#7752,#4728,.T.);
#9467=EDGE_CURVE('',#7759,#7754,#4729,.T.);
#9468=EDGE_CURVE('',#7760,#7761,#4730,.T.);
#9469=EDGE_CURVE('',#7762,#7760,#4731,.T.);
#9470=EDGE_CURVE('',#7762,#7763,#4732,.T.);
#9471=EDGE_CURVE('',#7763,#7761,#4733,.T.);
#9472=EDGE_CURVE('',#7761,#7764,#4734,.T.);
#9473=EDGE_CURVE('',#7763,#7765,#4735,.T.);
#9474=EDGE_CURVE('',#7765,#7764,#4736,.T.);
#9475=EDGE_CURVE('',#7764,#7766,#4737,.T.);
#9476=EDGE_CURVE('',#7765,#7767,#4738,.T.);
#9477=EDGE_CURVE('',#7767,#7766,#4739,.T.);
#9478=EDGE_CURVE('',#7766,#7760,#4740,.T.);
#9479=EDGE_CURVE('',#7767,#7762,#4741,.T.);
#9480=EDGE_CURVE('',#7768,#7769,#4742,.T.);
#9481=EDGE_CURVE('',#7770,#7768,#4743,.T.);
#9482=EDGE_CURVE('',#7770,#7771,#4744,.T.);
#9483=EDGE_CURVE('',#7771,#7769,#4745,.T.);
#9484=EDGE_CURVE('',#7769,#7772,#4746,.T.);
#9485=EDGE_CURVE('',#7771,#7773,#4747,.T.);
#9486=EDGE_CURVE('',#7773,#7772,#4748,.T.);
#9487=EDGE_CURVE('',#7772,#7774,#4749,.T.);
#9488=EDGE_CURVE('',#7773,#7775,#4750,.T.);
#9489=EDGE_CURVE('',#7775,#7774,#4751,.T.);
#9490=EDGE_CURVE('',#7774,#7768,#4752,.T.);
#9491=EDGE_CURVE('',#7775,#7770,#4753,.T.);
#9492=EDGE_CURVE('',#7776,#7777,#4754,.T.);
#9493=EDGE_CURVE('',#7778,#7776,#4755,.T.);
#9494=EDGE_CURVE('',#7778,#7779,#4756,.T.);
#9495=EDGE_CURVE('',#7779,#7777,#4757,.T.);
#9496=EDGE_CURVE('',#7777,#7780,#4758,.T.);
#9497=EDGE_CURVE('',#7779,#7781,#4759,.T.);
#9498=EDGE_CURVE('',#7781,#7780,#4760,.T.);
#9499=EDGE_CURVE('',#7780,#7782,#4761,.T.);
#9500=EDGE_CURVE('',#7781,#7783,#4762,.T.);
#9501=EDGE_CURVE('',#7783,#7782,#4763,.T.);
#9502=EDGE_CURVE('',#7782,#7776,#4764,.T.);
#9503=EDGE_CURVE('',#7783,#7778,#4765,.T.);
#9504=EDGE_CURVE('',#7784,#7784,#6873,.T.);
#9505=EDGE_CURVE('',#7784,#7785,#4766,.T.);
#9506=EDGE_CURVE('',#7785,#7785,#6874,.T.);
#9507=EDGE_CURVE('',#7786,#7786,#6875,.T.);
#9508=EDGE_CURVE('',#7786,#7787,#4767,.T.);
#9509=EDGE_CURVE('',#7787,#7787,#6876,.T.);
#9510=EDGE_CURVE('',#7788,#7788,#6877,.T.);
#9511=EDGE_CURVE('',#7788,#7789,#4768,.T.);
#9512=EDGE_CURVE('',#7789,#7789,#6878,.T.);
#9513=EDGE_CURVE('',#7790,#7791,#4769,.T.);
#9514=EDGE_CURVE('',#7792,#7790,#4770,.T.);
#9515=EDGE_CURVE('',#7792,#7793,#4771,.T.);
#9516=EDGE_CURVE('',#7791,#7793,#4772,.T.);
#9517=EDGE_CURVE('',#7794,#7795,#4773,.T.);
#9518=EDGE_CURVE('',#7796,#7794,#4774,.T.);
#9519=EDGE_CURVE('',#7797,#7796,#4775,.T.);
#9520=EDGE_CURVE('',#7795,#7797,#4776,.T.);
#9521=EDGE_CURVE('',#7797,#7798,#4777,.T.);
#9522=EDGE_CURVE('',#7799,#7796,#4778,.T.);
#9523=EDGE_CURVE('',#7798,#7799,#4779,.T.);
#9524=EDGE_CURVE('',#7798,#7800,#4780,.T.);
#9525=EDGE_CURVE('',#7801,#7799,#4781,.T.);
#9526=EDGE_CURVE('',#7800,#7801,#4782,.T.);
#9527=EDGE_CURVE('',#7800,#7792,#4783,.T.);
#9528=EDGE_CURVE('',#7793,#7801,#4784,.T.);
#9529=EDGE_CURVE('',#7802,#7795,#4785,.T.);
#9530=EDGE_CURVE('',#7803,#7802,#4786,.T.);
#9531=EDGE_CURVE('',#7794,#7803,#4787,.T.);
#9532=EDGE_CURVE('',#7790,#7804,#4788,.T.);
#9533=EDGE_CURVE('',#7802,#7804,#6879,.T.);
#9534=EDGE_CURVE('',#7805,#7791,#4789,.T.);
#9535=EDGE_CURVE('',#7804,#7805,#4790,.T.);
#9536=EDGE_CURVE('',#7803,#7805,#6880,.T.);
#11929=ORIENTED_EDGE('',*,*,#9216,.F.);
#11930=ORIENTED_EDGE('',*,*,#9217,.F.);
#11931=ORIENTED_EDGE('',*,*,#9218,.T.);
#11932=ORIENTED_EDGE('',*,*,#9219,.T.);
#11933=ORIENTED_EDGE('',*,*,#9220,.F.);
#11934=ORIENTED_EDGE('',*,*,#9219,.F.);
#11935=ORIENTED_EDGE('',*,*,#9221,.T.);
#11936=ORIENTED_EDGE('',*,*,#9222,.T.);
#11937=ORIENTED_EDGE('',*,*,#9223,.F.);
#11938=ORIENTED_EDGE('',*,*,#9222,.F.);
#11939=ORIENTED_EDGE('',*,*,#9224,.T.);
#11940=ORIENTED_EDGE('',*,*,#9225,.T.);
#11941=ORIENTED_EDGE('',*,*,#9226,.F.);
#11942=ORIENTED_EDGE('',*,*,#9225,.F.);
#11943=ORIENTED_EDGE('',*,*,#9227,.T.);
#11944=ORIENTED_EDGE('',*,*,#9217,.T.);
#11945=ORIENTED_EDGE('',*,*,#9221,.F.);
#11946=ORIENTED_EDGE('',*,*,#9218,.F.);
#11947=ORIENTED_EDGE('',*,*,#9227,.F.);
#11948=ORIENTED_EDGE('',*,*,#9224,.F.);
#11949=ORIENTED_EDGE('',*,*,#9228,.F.);
#11950=ORIENTED_EDGE('',*,*,#9229,.F.);
#11951=ORIENTED_EDGE('',*,*,#9230,.T.);
#11952=ORIENTED_EDGE('',*,*,#9231,.T.);
#11953=ORIENTED_EDGE('',*,*,#9232,.F.);
#11954=ORIENTED_EDGE('',*,*,#9231,.F.);
#11955=ORIENTED_EDGE('',*,*,#9233,.T.);
#11956=ORIENTED_EDGE('',*,*,#9234,.T.);
#11957=ORIENTED_EDGE('',*,*,#9235,.F.);
#11958=ORIENTED_EDGE('',*,*,#9234,.F.);
#11959=ORIENTED_EDGE('',*,*,#9236,.T.);
#11960=ORIENTED_EDGE('',*,*,#9237,.T.);
#11961=ORIENTED_EDGE('',*,*,#9238,.F.);
#11962=ORIENTED_EDGE('',*,*,#9237,.F.);
#11963=ORIENTED_EDGE('',*,*,#9239,.T.);
#11964=ORIENTED_EDGE('',*,*,#9229,.T.);
#11965=ORIENTED_EDGE('',*,*,#9233,.F.);
#11966=ORIENTED_EDGE('',*,*,#9230,.F.);
#11967=ORIENTED_EDGE('',*,*,#9239,.F.);
#11968=ORIENTED_EDGE('',*,*,#9236,.F.);
#11969=ORIENTED_EDGE('',*,*,#9240,.F.);
#11970=ORIENTED_EDGE('',*,*,#9241,.F.);
#11971=ORIENTED_EDGE('',*,*,#9242,.T.);
#11972=ORIENTED_EDGE('',*,*,#9243,.T.);
#11973=ORIENTED_EDGE('',*,*,#9244,.F.);
#11974=ORIENTED_EDGE('',*,*,#9243,.F.);
#11975=ORIENTED_EDGE('',*,*,#9245,.T.);
#11976=ORIENTED_EDGE('',*,*,#9246,.T.);
#11977=ORIENTED_EDGE('',*,*,#9247,.F.);
#11978=ORIENTED_EDGE('',*,*,#9246,.F.);
#11979=ORIENTED_EDGE('',*,*,#9248,.T.);
#11980=ORIENTED_EDGE('',*,*,#9249,.T.);
#11981=ORIENTED_EDGE('',*,*,#9250,.F.);
#11982=ORIENTED_EDGE('',*,*,#9249,.F.);
#11983=ORIENTED_EDGE('',*,*,#9251,.T.);
#11984=ORIENTED_EDGE('',*,*,#9241,.T.);
#11985=ORIENTED_EDGE('',*,*,#9245,.F.);
#11986=ORIENTED_EDGE('',*,*,#9242,.F.);
#11987=ORIENTED_EDGE('',*,*,#9251,.F.);
#11988=ORIENTED_EDGE('',*,*,#9248,.F.);
#11989=ORIENTED_EDGE('',*,*,#9252,.F.);
#11990=ORIENTED_EDGE('',*,*,#9253,.F.);
#11991=ORIENTED_EDGE('',*,*,#9254,.T.);
#11992=ORIENTED_EDGE('',*,*,#9255,.T.);
#11993=ORIENTED_EDGE('',*,*,#9256,.F.);
#11994=ORIENTED_EDGE('',*,*,#9255,.F.);
#11995=ORIENTED_EDGE('',*,*,#9257,.T.);
#11996=ORIENTED_EDGE('',*,*,#9258,.T.);
#11997=ORIENTED_EDGE('',*,*,#9259,.F.);
#11998=ORIENTED_EDGE('',*,*,#9258,.F.);
#11999=ORIENTED_EDGE('',*,*,#9260,.T.);
#12000=ORIENTED_EDGE('',*,*,#9261,.T.);
#12001=ORIENTED_EDGE('',*,*,#9262,.F.);
#12002=ORIENTED_EDGE('',*,*,#9261,.F.);
#12003=ORIENTED_EDGE('',*,*,#9263,.T.);
#12004=ORIENTED_EDGE('',*,*,#9253,.T.);
#12005=ORIENTED_EDGE('',*,*,#9257,.F.);
#12006=ORIENTED_EDGE('',*,*,#9254,.F.);
#12007=ORIENTED_EDGE('',*,*,#9263,.F.);
#12008=ORIENTED_EDGE('',*,*,#9260,.F.);
#12009=ORIENTED_EDGE('',*,*,#9264,.F.);
#12010=ORIENTED_EDGE('',*,*,#9265,.F.);
#12011=ORIENTED_EDGE('',*,*,#9266,.T.);
#12012=ORIENTED_EDGE('',*,*,#9267,.T.);
#12013=ORIENTED_EDGE('',*,*,#9268,.F.);
#12014=ORIENTED_EDGE('',*,*,#9267,.F.);
#12015=ORIENTED_EDGE('',*,*,#9269,.T.);
#12016=ORIENTED_EDGE('',*,*,#9270,.T.);
#12017=ORIENTED_EDGE('',*,*,#9271,.F.);
#12018=ORIENTED_EDGE('',*,*,#9270,.F.);
#12019=ORIENTED_EDGE('',*,*,#9272,.T.);
#12020=ORIENTED_EDGE('',*,*,#9273,.T.);
#12021=ORIENTED_EDGE('',*,*,#9274,.F.);
#12022=ORIENTED_EDGE('',*,*,#9273,.F.);
#12023=ORIENTED_EDGE('',*,*,#9275,.T.);
#12024=ORIENTED_EDGE('',*,*,#9265,.T.);
#12025=ORIENTED_EDGE('',*,*,#9269,.F.);
#12026=ORIENTED_EDGE('',*,*,#9266,.F.);
#12027=ORIENTED_EDGE('',*,*,#9275,.F.);
#12028=ORIENTED_EDGE('',*,*,#9272,.F.);
#12029=ORIENTED_EDGE('',*,*,#9276,.F.);
#12030=ORIENTED_EDGE('',*,*,#9277,.F.);
#12031=ORIENTED_EDGE('',*,*,#9278,.T.);
#12032=ORIENTED_EDGE('',*,*,#9279,.T.);
#12033=ORIENTED_EDGE('',*,*,#9280,.F.);
#12034=ORIENTED_EDGE('',*,*,#9279,.F.);
#12035=ORIENTED_EDGE('',*,*,#9281,.T.);
#12036=ORIENTED_EDGE('',*,*,#9282,.T.);
#12037=ORIENTED_EDGE('',*,*,#9283,.F.);
#12038=ORIENTED_EDGE('',*,*,#9282,.F.);
#12039=ORIENTED_EDGE('',*,*,#9284,.T.);
#12040=ORIENTED_EDGE('',*,*,#9285,.T.);
#12041=ORIENTED_EDGE('',*,*,#9286,.F.);
#12042=ORIENTED_EDGE('',*,*,#9285,.F.);
#12043=ORIENTED_EDGE('',*,*,#9287,.T.);
#12044=ORIENTED_EDGE('',*,*,#9277,.T.);
#12045=ORIENTED_EDGE('',*,*,#9281,.F.);
#12046=ORIENTED_EDGE('',*,*,#9278,.F.);
#12047=ORIENTED_EDGE('',*,*,#9287,.F.);
#12048=ORIENTED_EDGE('',*,*,#9284,.F.);
#12049=ORIENTED_EDGE('',*,*,#9288,.F.);
#12050=ORIENTED_EDGE('',*,*,#9289,.F.);
#12051=ORIENTED_EDGE('',*,*,#9290,.T.);
#12052=ORIENTED_EDGE('',*,*,#9291,.T.);
#12053=ORIENTED_EDGE('',*,*,#9292,.F.);
#12054=ORIENTED_EDGE('',*,*,#9291,.F.);
#12055=ORIENTED_EDGE('',*,*,#9293,.T.);
#12056=ORIENTED_EDGE('',*,*,#9294,.T.);
#12057=ORIENTED_EDGE('',*,*,#9295,.F.);
#12058=ORIENTED_EDGE('',*,*,#9294,.F.);
#12059=ORIENTED_EDGE('',*,*,#9296,.T.);
#12060=ORIENTED_EDGE('',*,*,#9297,.T.);
#12061=ORIENTED_EDGE('',*,*,#9298,.F.);
#12062=ORIENTED_EDGE('',*,*,#9297,.F.);
#12063=ORIENTED_EDGE('',*,*,#9299,.T.);
#12064=ORIENTED_EDGE('',*,*,#9289,.T.);
#12065=ORIENTED_EDGE('',*,*,#9293,.F.);
#12066=ORIENTED_EDGE('',*,*,#9290,.F.);
#12067=ORIENTED_EDGE('',*,*,#9299,.F.);
#12068=ORIENTED_EDGE('',*,*,#9296,.F.);
#12069=ORIENTED_EDGE('',*,*,#9300,.F.);
#12070=ORIENTED_EDGE('',*,*,#9301,.F.);
#12071=ORIENTED_EDGE('',*,*,#9302,.T.);
#12072=ORIENTED_EDGE('',*,*,#9303,.T.);
#12073=ORIENTED_EDGE('',*,*,#9304,.F.);
#12074=ORIENTED_EDGE('',*,*,#9303,.F.);
#12075=ORIENTED_EDGE('',*,*,#9305,.T.);
#12076=ORIENTED_EDGE('',*,*,#9306,.T.);
#12077=ORIENTED_EDGE('',*,*,#9307,.F.);
#12078=ORIENTED_EDGE('',*,*,#9306,.F.);
#12079=ORIENTED_EDGE('',*,*,#9308,.T.);
#12080=ORIENTED_EDGE('',*,*,#9309,.T.);
#12081=ORIENTED_EDGE('',*,*,#9310,.F.);
#12082=ORIENTED_EDGE('',*,*,#9309,.F.);
#12083=ORIENTED_EDGE('',*,*,#9311,.T.);
#12084=ORIENTED_EDGE('',*,*,#9301,.T.);
#12085=ORIENTED_EDGE('',*,*,#9305,.F.);
#12086=ORIENTED_EDGE('',*,*,#9302,.F.);
#12087=ORIENTED_EDGE('',*,*,#9311,.F.);
#12088=ORIENTED_EDGE('',*,*,#9308,.F.);
#12089=ORIENTED_EDGE('',*,*,#9312,.F.);
#12090=ORIENTED_EDGE('',*,*,#9313,.F.);
#12091=ORIENTED_EDGE('',*,*,#9314,.T.);
#12092=ORIENTED_EDGE('',*,*,#9315,.T.);
#12093=ORIENTED_EDGE('',*,*,#9316,.F.);
#12094=ORIENTED_EDGE('',*,*,#9315,.F.);
#12095=ORIENTED_EDGE('',*,*,#9317,.T.);
#12096=ORIENTED_EDGE('',*,*,#9318,.T.);
#12097=ORIENTED_EDGE('',*,*,#9319,.F.);
#12098=ORIENTED_EDGE('',*,*,#9318,.F.);
#12099=ORIENTED_EDGE('',*,*,#9320,.T.);
#12100=ORIENTED_EDGE('',*,*,#9321,.T.);
#12101=ORIENTED_EDGE('',*,*,#9322,.F.);
#12102=ORIENTED_EDGE('',*,*,#9321,.F.);
#12103=ORIENTED_EDGE('',*,*,#9323,.T.);
#12104=ORIENTED_EDGE('',*,*,#9313,.T.);
#12105=ORIENTED_EDGE('',*,*,#9317,.F.);
#12106=ORIENTED_EDGE('',*,*,#9314,.F.);
#12107=ORIENTED_EDGE('',*,*,#9323,.F.);
#12108=ORIENTED_EDGE('',*,*,#9320,.F.);
#12109=ORIENTED_EDGE('',*,*,#9324,.F.);
#12110=ORIENTED_EDGE('',*,*,#9325,.F.);
#12111=ORIENTED_EDGE('',*,*,#9326,.T.);
#12112=ORIENTED_EDGE('',*,*,#9327,.T.);
#12113=ORIENTED_EDGE('',*,*,#9328,.F.);
#12114=ORIENTED_EDGE('',*,*,#9327,.F.);
#12115=ORIENTED_EDGE('',*,*,#9329,.T.);
#12116=ORIENTED_EDGE('',*,*,#9330,.T.);
#12117=ORIENTED_EDGE('',*,*,#9331,.F.);
#12118=ORIENTED_EDGE('',*,*,#9330,.F.);
#12119=ORIENTED_EDGE('',*,*,#9332,.T.);
#12120=ORIENTED_EDGE('',*,*,#9333,.T.);
#12121=ORIENTED_EDGE('',*,*,#9334,.F.);
#12122=ORIENTED_EDGE('',*,*,#9333,.F.);
#12123=ORIENTED_EDGE('',*,*,#9335,.T.);
#12124=ORIENTED_EDGE('',*,*,#9325,.T.);
#12125=ORIENTED_EDGE('',*,*,#9329,.F.);
#12126=ORIENTED_EDGE('',*,*,#9326,.F.);
#12127=ORIENTED_EDGE('',*,*,#9335,.F.);
#12128=ORIENTED_EDGE('',*,*,#9332,.F.);
#12129=ORIENTED_EDGE('',*,*,#9336,.F.);
#12130=ORIENTED_EDGE('',*,*,#9337,.F.);
#12131=ORIENTED_EDGE('',*,*,#9338,.T.);
#12132=ORIENTED_EDGE('',*,*,#9339,.T.);
#12133=ORIENTED_EDGE('',*,*,#9340,.F.);
#12134=ORIENTED_EDGE('',*,*,#9339,.F.);
#12135=ORIENTED_EDGE('',*,*,#9341,.T.);
#12136=ORIENTED_EDGE('',*,*,#9342,.T.);
#12137=ORIENTED_EDGE('',*,*,#9343,.F.);
#12138=ORIENTED_EDGE('',*,*,#9342,.F.);
#12139=ORIENTED_EDGE('',*,*,#9344,.T.);
#12140=ORIENTED_EDGE('',*,*,#9345,.T.);
#12141=ORIENTED_EDGE('',*,*,#9346,.F.);
#12142=ORIENTED_EDGE('',*,*,#9345,.F.);
#12143=ORIENTED_EDGE('',*,*,#9347,.T.);
#12144=ORIENTED_EDGE('',*,*,#9337,.T.);
#12145=ORIENTED_EDGE('',*,*,#9341,.F.);
#12146=ORIENTED_EDGE('',*,*,#9338,.F.);
#12147=ORIENTED_EDGE('',*,*,#9347,.F.);
#12148=ORIENTED_EDGE('',*,*,#9344,.F.);
#12149=ORIENTED_EDGE('',*,*,#9348,.F.);
#12150=ORIENTED_EDGE('',*,*,#9349,.F.);
#12151=ORIENTED_EDGE('',*,*,#9350,.T.);
#12152=ORIENTED_EDGE('',*,*,#9351,.T.);
#12153=ORIENTED_EDGE('',*,*,#9352,.F.);
#12154=ORIENTED_EDGE('',*,*,#9351,.F.);
#12155=ORIENTED_EDGE('',*,*,#9353,.T.);
#12156=ORIENTED_EDGE('',*,*,#9354,.T.);
#12157=ORIENTED_EDGE('',*,*,#9355,.F.);
#12158=ORIENTED_EDGE('',*,*,#9354,.F.);
#12159=ORIENTED_EDGE('',*,*,#9356,.T.);
#12160=ORIENTED_EDGE('',*,*,#9357,.T.);
#12161=ORIENTED_EDGE('',*,*,#9358,.F.);
#12162=ORIENTED_EDGE('',*,*,#9357,.F.);
#12163=ORIENTED_EDGE('',*,*,#9359,.T.);
#12164=ORIENTED_EDGE('',*,*,#9349,.T.);
#12165=ORIENTED_EDGE('',*,*,#9353,.F.);
#12166=ORIENTED_EDGE('',*,*,#9350,.F.);
#12167=ORIENTED_EDGE('',*,*,#9359,.F.);
#12168=ORIENTED_EDGE('',*,*,#9356,.F.);
#12169=ORIENTED_EDGE('',*,*,#9360,.F.);
#12170=ORIENTED_EDGE('',*,*,#9361,.F.);
#12171=ORIENTED_EDGE('',*,*,#9362,.T.);
#12172=ORIENTED_EDGE('',*,*,#9363,.T.);
#12173=ORIENTED_EDGE('',*,*,#9364,.F.);
#12174=ORIENTED_EDGE('',*,*,#9363,.F.);
#12175=ORIENTED_EDGE('',*,*,#9365,.T.);
#12176=ORIENTED_EDGE('',*,*,#9366,.T.);
#12177=ORIENTED_EDGE('',*,*,#9367,.F.);
#12178=ORIENTED_EDGE('',*,*,#9366,.F.);
#12179=ORIENTED_EDGE('',*,*,#9368,.T.);
#12180=ORIENTED_EDGE('',*,*,#9369,.T.);
#12181=ORIENTED_EDGE('',*,*,#9370,.F.);
#12182=ORIENTED_EDGE('',*,*,#9369,.F.);
#12183=ORIENTED_EDGE('',*,*,#9371,.T.);
#12184=ORIENTED_EDGE('',*,*,#9361,.T.);
#12185=ORIENTED_EDGE('',*,*,#9365,.F.);
#12186=ORIENTED_EDGE('',*,*,#9362,.F.);
#12187=ORIENTED_EDGE('',*,*,#9371,.F.);
#12188=ORIENTED_EDGE('',*,*,#9368,.F.);
#12189=ORIENTED_EDGE('',*,*,#9372,.F.);
#12190=ORIENTED_EDGE('',*,*,#9373,.F.);
#12191=ORIENTED_EDGE('',*,*,#9374,.T.);
#12192=ORIENTED_EDGE('',*,*,#9375,.T.);
#12193=ORIENTED_EDGE('',*,*,#9376,.F.);
#12194=ORIENTED_EDGE('',*,*,#9375,.F.);
#12195=ORIENTED_EDGE('',*,*,#9377,.T.);
#12196=ORIENTED_EDGE('',*,*,#9378,.T.);
#12197=ORIENTED_EDGE('',*,*,#9379,.F.);
#12198=ORIENTED_EDGE('',*,*,#9378,.F.);
#12199=ORIENTED_EDGE('',*,*,#9380,.T.);
#12200=ORIENTED_EDGE('',*,*,#9381,.T.);
#12201=ORIENTED_EDGE('',*,*,#9382,.F.);
#12202=ORIENTED_EDGE('',*,*,#9381,.F.);
#12203=ORIENTED_EDGE('',*,*,#9383,.T.);
#12204=ORIENTED_EDGE('',*,*,#9373,.T.);
#12205=ORIENTED_EDGE('',*,*,#9377,.F.);
#12206=ORIENTED_EDGE('',*,*,#9374,.F.);
#12207=ORIENTED_EDGE('',*,*,#9383,.F.);
#12208=ORIENTED_EDGE('',*,*,#9380,.F.);
#12209=ORIENTED_EDGE('',*,*,#9384,.F.);
#12210=ORIENTED_EDGE('',*,*,#9385,.F.);
#12211=ORIENTED_EDGE('',*,*,#9386,.T.);
#12212=ORIENTED_EDGE('',*,*,#9387,.T.);
#12213=ORIENTED_EDGE('',*,*,#9388,.F.);
#12214=ORIENTED_EDGE('',*,*,#9387,.F.);
#12215=ORIENTED_EDGE('',*,*,#9389,.T.);
#12216=ORIENTED_EDGE('',*,*,#9390,.T.);
#12217=ORIENTED_EDGE('',*,*,#9391,.F.);
#12218=ORIENTED_EDGE('',*,*,#9390,.F.);
#12219=ORIENTED_EDGE('',*,*,#9392,.T.);
#12220=ORIENTED_EDGE('',*,*,#9393,.T.);
#12221=ORIENTED_EDGE('',*,*,#9394,.F.);
#12222=ORIENTED_EDGE('',*,*,#9393,.F.);
#12223=ORIENTED_EDGE('',*,*,#9395,.T.);
#12224=ORIENTED_EDGE('',*,*,#9385,.T.);
#12225=ORIENTED_EDGE('',*,*,#9389,.F.);
#12226=ORIENTED_EDGE('',*,*,#9386,.F.);
#12227=ORIENTED_EDGE('',*,*,#9395,.F.);
#12228=ORIENTED_EDGE('',*,*,#9392,.F.);
#12229=ORIENTED_EDGE('',*,*,#9396,.F.);
#12230=ORIENTED_EDGE('',*,*,#9397,.F.);
#12231=ORIENTED_EDGE('',*,*,#9398,.T.);
#12232=ORIENTED_EDGE('',*,*,#9399,.T.);
#12233=ORIENTED_EDGE('',*,*,#9400,.F.);
#12234=ORIENTED_EDGE('',*,*,#9399,.F.);
#12235=ORIENTED_EDGE('',*,*,#9401,.T.);
#12236=ORIENTED_EDGE('',*,*,#9402,.T.);
#12237=ORIENTED_EDGE('',*,*,#9403,.F.);
#12238=ORIENTED_EDGE('',*,*,#9402,.F.);
#12239=ORIENTED_EDGE('',*,*,#9404,.T.);
#12240=ORIENTED_EDGE('',*,*,#9405,.T.);
#12241=ORIENTED_EDGE('',*,*,#9406,.F.);
#12242=ORIENTED_EDGE('',*,*,#9405,.F.);
#12243=ORIENTED_EDGE('',*,*,#9407,.T.);
#12244=ORIENTED_EDGE('',*,*,#9397,.T.);
#12245=ORIENTED_EDGE('',*,*,#9401,.F.);
#12246=ORIENTED_EDGE('',*,*,#9398,.F.);
#12247=ORIENTED_EDGE('',*,*,#9407,.F.);
#12248=ORIENTED_EDGE('',*,*,#9404,.F.);
#12249=ORIENTED_EDGE('',*,*,#9408,.F.);
#12250=ORIENTED_EDGE('',*,*,#9409,.F.);
#12251=ORIENTED_EDGE('',*,*,#9410,.T.);
#12252=ORIENTED_EDGE('',*,*,#9411,.T.);
#12253=ORIENTED_EDGE('',*,*,#9412,.F.);
#12254=ORIENTED_EDGE('',*,*,#9411,.F.);
#12255=ORIENTED_EDGE('',*,*,#9413,.T.);
#12256=ORIENTED_EDGE('',*,*,#9414,.T.);
#12257=ORIENTED_EDGE('',*,*,#9415,.F.);
#12258=ORIENTED_EDGE('',*,*,#9414,.F.);
#12259=ORIENTED_EDGE('',*,*,#9416,.T.);
#12260=ORIENTED_EDGE('',*,*,#9417,.T.);
#12261=ORIENTED_EDGE('',*,*,#9418,.F.);
#12262=ORIENTED_EDGE('',*,*,#9417,.F.);
#12263=ORIENTED_EDGE('',*,*,#9419,.T.);
#12264=ORIENTED_EDGE('',*,*,#9409,.T.);
#12265=ORIENTED_EDGE('',*,*,#9413,.F.);
#12266=ORIENTED_EDGE('',*,*,#9410,.F.);
#12267=ORIENTED_EDGE('',*,*,#9419,.F.);
#12268=ORIENTED_EDGE('',*,*,#9416,.F.);
#12269=ORIENTED_EDGE('',*,*,#9420,.F.);
#12270=ORIENTED_EDGE('',*,*,#9421,.F.);
#12271=ORIENTED_EDGE('',*,*,#9422,.T.);
#12272=ORIENTED_EDGE('',*,*,#9423,.T.);
#12273=ORIENTED_EDGE('',*,*,#9424,.F.);
#12274=ORIENTED_EDGE('',*,*,#9423,.F.);
#12275=ORIENTED_EDGE('',*,*,#9425,.T.);
#12276=ORIENTED_EDGE('',*,*,#9426,.T.);
#12277=ORIENTED_EDGE('',*,*,#9427,.F.);
#12278=ORIENTED_EDGE('',*,*,#9426,.F.);
#12279=ORIENTED_EDGE('',*,*,#9428,.T.);
#12280=ORIENTED_EDGE('',*,*,#9429,.T.);
#12281=ORIENTED_EDGE('',*,*,#9430,.F.);
#12282=ORIENTED_EDGE('',*,*,#9429,.F.);
#12283=ORIENTED_EDGE('',*,*,#9431,.T.);
#12284=ORIENTED_EDGE('',*,*,#9421,.T.);
#12285=ORIENTED_EDGE('',*,*,#9425,.F.);
#12286=ORIENTED_EDGE('',*,*,#9422,.F.);
#12287=ORIENTED_EDGE('',*,*,#9431,.F.);
#12288=ORIENTED_EDGE('',*,*,#9428,.F.);
#12289=ORIENTED_EDGE('',*,*,#9432,.F.);
#12290=ORIENTED_EDGE('',*,*,#9433,.F.);
#12291=ORIENTED_EDGE('',*,*,#9434,.T.);
#12292=ORIENTED_EDGE('',*,*,#9435,.T.);
#12293=ORIENTED_EDGE('',*,*,#9436,.F.);
#12294=ORIENTED_EDGE('',*,*,#9435,.F.);
#12295=ORIENTED_EDGE('',*,*,#9437,.T.);
#12296=ORIENTED_EDGE('',*,*,#9438,.T.);
#12297=ORIENTED_EDGE('',*,*,#9439,.F.);
#12298=ORIENTED_EDGE('',*,*,#9438,.F.);
#12299=ORIENTED_EDGE('',*,*,#9440,.T.);
#12300=ORIENTED_EDGE('',*,*,#9441,.T.);
#12301=ORIENTED_EDGE('',*,*,#9442,.F.);
#12302=ORIENTED_EDGE('',*,*,#9441,.F.);
#12303=ORIENTED_EDGE('',*,*,#9443,.T.);
#12304=ORIENTED_EDGE('',*,*,#9433,.T.);
#12305=ORIENTED_EDGE('',*,*,#9437,.F.);
#12306=ORIENTED_EDGE('',*,*,#9434,.F.);
#12307=ORIENTED_EDGE('',*,*,#9443,.F.);
#12308=ORIENTED_EDGE('',*,*,#9440,.F.);
#12309=ORIENTED_EDGE('',*,*,#9444,.F.);
#12310=ORIENTED_EDGE('',*,*,#9445,.F.);
#12311=ORIENTED_EDGE('',*,*,#9446,.T.);
#12312=ORIENTED_EDGE('',*,*,#9447,.T.);
#12313=ORIENTED_EDGE('',*,*,#9448,.F.);
#12314=ORIENTED_EDGE('',*,*,#9447,.F.);
#12315=ORIENTED_EDGE('',*,*,#9449,.T.);
#12316=ORIENTED_EDGE('',*,*,#9450,.T.);
#12317=ORIENTED_EDGE('',*,*,#9451,.F.);
#12318=ORIENTED_EDGE('',*,*,#9450,.F.);
#12319=ORIENTED_EDGE('',*,*,#9452,.T.);
#12320=ORIENTED_EDGE('',*,*,#9453,.T.);
#12321=ORIENTED_EDGE('',*,*,#9454,.F.);
#12322=ORIENTED_EDGE('',*,*,#9453,.F.);
#12323=ORIENTED_EDGE('',*,*,#9455,.T.);
#12324=ORIENTED_EDGE('',*,*,#9445,.T.);
#12325=ORIENTED_EDGE('',*,*,#9449,.F.);
#12326=ORIENTED_EDGE('',*,*,#9446,.F.);
#12327=ORIENTED_EDGE('',*,*,#9455,.F.);
#12328=ORIENTED_EDGE('',*,*,#9452,.F.);
#12329=ORIENTED_EDGE('',*,*,#9456,.F.);
#12330=ORIENTED_EDGE('',*,*,#9457,.F.);
#12331=ORIENTED_EDGE('',*,*,#9458,.T.);
#12332=ORIENTED_EDGE('',*,*,#9459,.T.);
#12333=ORIENTED_EDGE('',*,*,#9460,.F.);
#12334=ORIENTED_EDGE('',*,*,#9459,.F.);
#12335=ORIENTED_EDGE('',*,*,#9461,.T.);
#12336=ORIENTED_EDGE('',*,*,#9462,.T.);
#12337=ORIENTED_EDGE('',*,*,#9463,.F.);
#12338=ORIENTED_EDGE('',*,*,#9462,.F.);
#12339=ORIENTED_EDGE('',*,*,#9464,.T.);
#12340=ORIENTED_EDGE('',*,*,#9465,.T.);
#12341=ORIENTED_EDGE('',*,*,#9466,.F.);
#12342=ORIENTED_EDGE('',*,*,#9465,.F.);
#12343=ORIENTED_EDGE('',*,*,#9467,.T.);
#12344=ORIENTED_EDGE('',*,*,#9457,.T.);
#12345=ORIENTED_EDGE('',*,*,#9461,.F.);
#12346=ORIENTED_EDGE('',*,*,#9458,.F.);
#12347=ORIENTED_EDGE('',*,*,#9467,.F.);
#12348=ORIENTED_EDGE('',*,*,#9464,.F.);
#12349=ORIENTED_EDGE('',*,*,#9468,.F.);
#12350=ORIENTED_EDGE('',*,*,#9469,.F.);
#12351=ORIENTED_EDGE('',*,*,#9470,.T.);
#12352=ORIENTED_EDGE('',*,*,#9471,.T.);
#12353=ORIENTED_EDGE('',*,*,#9472,.F.);
#12354=ORIENTED_EDGE('',*,*,#9471,.F.);
#12355=ORIENTED_EDGE('',*,*,#9473,.T.);
#12356=ORIENTED_EDGE('',*,*,#9474,.T.);
#12357=ORIENTED_EDGE('',*,*,#9475,.F.);
#12358=ORIENTED_EDGE('',*,*,#9474,.F.);
#12359=ORIENTED_EDGE('',*,*,#9476,.T.);
#12360=ORIENTED_EDGE('',*,*,#9477,.T.);
#12361=ORIENTED_EDGE('',*,*,#9478,.F.);
#12362=ORIENTED_EDGE('',*,*,#9477,.F.);
#12363=ORIENTED_EDGE('',*,*,#9479,.T.);
#12364=ORIENTED_EDGE('',*,*,#9469,.T.);
#12365=ORIENTED_EDGE('',*,*,#9473,.F.);
#12366=ORIENTED_EDGE('',*,*,#9470,.F.);
#12367=ORIENTED_EDGE('',*,*,#9479,.F.);
#12368=ORIENTED_EDGE('',*,*,#9476,.F.);
#12369=ORIENTED_EDGE('',*,*,#9480,.F.);
#12370=ORIENTED_EDGE('',*,*,#9481,.F.);
#12371=ORIENTED_EDGE('',*,*,#9482,.T.);
#12372=ORIENTED_EDGE('',*,*,#9483,.T.);
#12373=ORIENTED_EDGE('',*,*,#9484,.F.);
#12374=ORIENTED_EDGE('',*,*,#9483,.F.);
#12375=ORIENTED_EDGE('',*,*,#9485,.T.);
#12376=ORIENTED_EDGE('',*,*,#9486,.T.);
#12377=ORIENTED_EDGE('',*,*,#9487,.F.);
#12378=ORIENTED_EDGE('',*,*,#9486,.F.);
#12379=ORIENTED_EDGE('',*,*,#9488,.T.);
#12380=ORIENTED_EDGE('',*,*,#9489,.T.);
#12381=ORIENTED_EDGE('',*,*,#9490,.F.);
#12382=ORIENTED_EDGE('',*,*,#9489,.F.);
#12383=ORIENTED_EDGE('',*,*,#9491,.T.);
#12384=ORIENTED_EDGE('',*,*,#9481,.T.);
#12385=ORIENTED_EDGE('',*,*,#9485,.F.);
#12386=ORIENTED_EDGE('',*,*,#9482,.F.);
#12387=ORIENTED_EDGE('',*,*,#9491,.F.);
#12388=ORIENTED_EDGE('',*,*,#9488,.F.);
#12389=ORIENTED_EDGE('',*,*,#9492,.F.);
#12390=ORIENTED_EDGE('',*,*,#9493,.F.);
#12391=ORIENTED_EDGE('',*,*,#9494,.T.);
#12392=ORIENTED_EDGE('',*,*,#9495,.T.);
#12393=ORIENTED_EDGE('',*,*,#9496,.F.);
#12394=ORIENTED_EDGE('',*,*,#9495,.F.);
#12395=ORIENTED_EDGE('',*,*,#9497,.T.);
#12396=ORIENTED_EDGE('',*,*,#9498,.T.);
#12397=ORIENTED_EDGE('',*,*,#9499,.F.);
#12398=ORIENTED_EDGE('',*,*,#9498,.F.);
#12399=ORIENTED_EDGE('',*,*,#9500,.T.);
#12400=ORIENTED_EDGE('',*,*,#9501,.T.);
#12401=ORIENTED_EDGE('',*,*,#9502,.F.);
#12402=ORIENTED_EDGE('',*,*,#9501,.F.);
#12403=ORIENTED_EDGE('',*,*,#9503,.T.);
#12404=ORIENTED_EDGE('',*,*,#9493,.T.);
#12405=ORIENTED_EDGE('',*,*,#9497,.F.);
#12406=ORIENTED_EDGE('',*,*,#9494,.F.);
#12407=ORIENTED_EDGE('',*,*,#9503,.F.);
#12408=ORIENTED_EDGE('',*,*,#9500,.F.);
#12409=ORIENTED_EDGE('',*,*,#9504,.F.);
#12410=ORIENTED_EDGE('',*,*,#9505,.T.);
#12411=ORIENTED_EDGE('',*,*,#9506,.F.);
#12412=ORIENTED_EDGE('',*,*,#9505,.F.);
#12413=ORIENTED_EDGE('',*,*,#9507,.F.);
#12414=ORIENTED_EDGE('',*,*,#9508,.T.);
#12415=ORIENTED_EDGE('',*,*,#9509,.F.);
#12416=ORIENTED_EDGE('',*,*,#9508,.F.);
#12417=ORIENTED_EDGE('',*,*,#9510,.F.);
#12418=ORIENTED_EDGE('',*,*,#9511,.T.);
#12419=ORIENTED_EDGE('',*,*,#9512,.F.);
#12420=ORIENTED_EDGE('',*,*,#9511,.F.);
#12421=ORIENTED_EDGE('',*,*,#9513,.F.);
#12422=ORIENTED_EDGE('',*,*,#9514,.F.);
#12423=ORIENTED_EDGE('',*,*,#9515,.T.);
#12424=ORIENTED_EDGE('',*,*,#9516,.F.);
#12425=ORIENTED_EDGE('',*,*,#9517,.F.);
#12426=ORIENTED_EDGE('',*,*,#9518,.F.);
#12427=ORIENTED_EDGE('',*,*,#9519,.F.);
#12428=ORIENTED_EDGE('',*,*,#9520,.F.);
#12429=ORIENTED_EDGE('',*,*,#9521,.F.);
#12430=ORIENTED_EDGE('',*,*,#9519,.T.);
#12431=ORIENTED_EDGE('',*,*,#9522,.F.);
#12432=ORIENTED_EDGE('',*,*,#9523,.F.);
#12433=ORIENTED_EDGE('',*,*,#9524,.F.);
#12434=ORIENTED_EDGE('',*,*,#9523,.T.);
#12435=ORIENTED_EDGE('',*,*,#9525,.F.);
#12436=ORIENTED_EDGE('',*,*,#9526,.F.);
#12437=ORIENTED_EDGE('',*,*,#9527,.F.);
#12438=ORIENTED_EDGE('',*,*,#9526,.T.);
#12439=ORIENTED_EDGE('',*,*,#9528,.F.);
#12440=ORIENTED_EDGE('',*,*,#9515,.F.);
#12441=ORIENTED_EDGE('',*,*,#9517,.T.);
#12442=ORIENTED_EDGE('',*,*,#9529,.F.);
#12443=ORIENTED_EDGE('',*,*,#9530,.F.);
#12444=ORIENTED_EDGE('',*,*,#9531,.F.);
#12445=ORIENTED_EDGE('',*,*,#9520,.T.);
#12446=ORIENTED_EDGE('',*,*,#9521,.T.);
#12447=ORIENTED_EDGE('',*,*,#9524,.T.);
#12448=ORIENTED_EDGE('',*,*,#9527,.T.);
#12449=ORIENTED_EDGE('',*,*,#9514,.T.);
#12450=ORIENTED_EDGE('',*,*,#9532,.T.);
#12451=ORIENTED_EDGE('',*,*,#9533,.F.);
#12452=ORIENTED_EDGE('',*,*,#9529,.T.);
#12453=ORIENTED_EDGE('',*,*,#9504,.T.);
#12454=ORIENTED_EDGE('',*,*,#9507,.T.);
#12455=ORIENTED_EDGE('',*,*,#9510,.T.);
#12456=ORIENTED_EDGE('',*,*,#9513,.T.);
#12457=ORIENTED_EDGE('',*,*,#9534,.F.);
#12458=ORIENTED_EDGE('',*,*,#9535,.F.);
#12459=ORIENTED_EDGE('',*,*,#9532,.F.);
#12460=ORIENTED_EDGE('',*,*,#9531,.T.);
#12461=ORIENTED_EDGE('',*,*,#9536,.T.);
#12462=ORIENTED_EDGE('',*,*,#9534,.T.);
#12463=ORIENTED_EDGE('',*,*,#9516,.T.);
#12464=ORIENTED_EDGE('',*,*,#9528,.T.);
#12465=ORIENTED_EDGE('',*,*,#9525,.T.);
#12466=ORIENTED_EDGE('',*,*,#9522,.T.);
#12467=ORIENTED_EDGE('',*,*,#9518,.T.);
#12468=ORIENTED_EDGE('',*,*,#9235,.T.);
#12469=ORIENTED_EDGE('',*,*,#9238,.T.);
#12470=ORIENTED_EDGE('',*,*,#9228,.T.);
#12471=ORIENTED_EDGE('',*,*,#9232,.T.);
#12472=ORIENTED_EDGE('',*,*,#9259,.T.);
#12473=ORIENTED_EDGE('',*,*,#9262,.T.);
#12474=ORIENTED_EDGE('',*,*,#9252,.T.);
#12475=ORIENTED_EDGE('',*,*,#9256,.T.);
#12476=ORIENTED_EDGE('',*,*,#9283,.T.);
#12477=ORIENTED_EDGE('',*,*,#9286,.T.);
#12478=ORIENTED_EDGE('',*,*,#9276,.T.);
#12479=ORIENTED_EDGE('',*,*,#9280,.T.);
#12480=ORIENTED_EDGE('',*,*,#9307,.T.);
#12481=ORIENTED_EDGE('',*,*,#9310,.T.);
#12482=ORIENTED_EDGE('',*,*,#9300,.T.);
#12483=ORIENTED_EDGE('',*,*,#9304,.T.);
#12484=ORIENTED_EDGE('',*,*,#9331,.T.);
#12485=ORIENTED_EDGE('',*,*,#9334,.T.);
#12486=ORIENTED_EDGE('',*,*,#9324,.T.);
#12487=ORIENTED_EDGE('',*,*,#9328,.T.);
#12488=ORIENTED_EDGE('',*,*,#9355,.T.);
#12489=ORIENTED_EDGE('',*,*,#9358,.T.);
#12490=ORIENTED_EDGE('',*,*,#9348,.T.);
#12491=ORIENTED_EDGE('',*,*,#9352,.T.);
#12492=ORIENTED_EDGE('',*,*,#9379,.T.);
#12493=ORIENTED_EDGE('',*,*,#9382,.T.);
#12494=ORIENTED_EDGE('',*,*,#9372,.T.);
#12495=ORIENTED_EDGE('',*,*,#9376,.T.);
#12496=ORIENTED_EDGE('',*,*,#9403,.T.);
#12497=ORIENTED_EDGE('',*,*,#9406,.T.);
#12498=ORIENTED_EDGE('',*,*,#9396,.T.);
#12499=ORIENTED_EDGE('',*,*,#9400,.T.);
#12500=ORIENTED_EDGE('',*,*,#9427,.T.);
#12501=ORIENTED_EDGE('',*,*,#9430,.T.);
#12502=ORIENTED_EDGE('',*,*,#9420,.T.);
#12503=ORIENTED_EDGE('',*,*,#9424,.T.);
#12504=ORIENTED_EDGE('',*,*,#9451,.T.);
#12505=ORIENTED_EDGE('',*,*,#9454,.T.);
#12506=ORIENTED_EDGE('',*,*,#9444,.T.);
#12507=ORIENTED_EDGE('',*,*,#9448,.T.);
#12508=ORIENTED_EDGE('',*,*,#9463,.T.);
#12509=ORIENTED_EDGE('',*,*,#9466,.T.);
#12510=ORIENTED_EDGE('',*,*,#9456,.T.);
#12511=ORIENTED_EDGE('',*,*,#9460,.T.);
#12512=ORIENTED_EDGE('',*,*,#9475,.T.);
#12513=ORIENTED_EDGE('',*,*,#9478,.T.);
#12514=ORIENTED_EDGE('',*,*,#9468,.T.);
#12515=ORIENTED_EDGE('',*,*,#9472,.T.);
#12516=ORIENTED_EDGE('',*,*,#9487,.T.);
#12517=ORIENTED_EDGE('',*,*,#9490,.T.);
#12518=ORIENTED_EDGE('',*,*,#9480,.T.);
#12519=ORIENTED_EDGE('',*,*,#9484,.T.);
#12520=ORIENTED_EDGE('',*,*,#9499,.T.);
#12521=ORIENTED_EDGE('',*,*,#9502,.T.);
#12522=ORIENTED_EDGE('',*,*,#9492,.T.);
#12523=ORIENTED_EDGE('',*,*,#9496,.T.);
#12524=ORIENTED_EDGE('',*,*,#9506,.T.);
#12525=ORIENTED_EDGE('',*,*,#9509,.T.);
#12526=ORIENTED_EDGE('',*,*,#9512,.T.);
#12527=ORIENTED_EDGE('',*,*,#9439,.T.);
#12528=ORIENTED_EDGE('',*,*,#9442,.T.);
#12529=ORIENTED_EDGE('',*,*,#9432,.T.);
#12530=ORIENTED_EDGE('',*,*,#9436,.T.);
#12531=ORIENTED_EDGE('',*,*,#9415,.T.);
#12532=ORIENTED_EDGE('',*,*,#9418,.T.);
#12533=ORIENTED_EDGE('',*,*,#9408,.T.);
#12534=ORIENTED_EDGE('',*,*,#9412,.T.);
#12535=ORIENTED_EDGE('',*,*,#9391,.T.);
#12536=ORIENTED_EDGE('',*,*,#9394,.T.);
#12537=ORIENTED_EDGE('',*,*,#9384,.T.);
#12538=ORIENTED_EDGE('',*,*,#9388,.T.);
#12539=ORIENTED_EDGE('',*,*,#9367,.T.);
#12540=ORIENTED_EDGE('',*,*,#9370,.T.);
#12541=ORIENTED_EDGE('',*,*,#9360,.T.);
#12542=ORIENTED_EDGE('',*,*,#9364,.T.);
#12543=ORIENTED_EDGE('',*,*,#9343,.T.);
#12544=ORIENTED_EDGE('',*,*,#9346,.T.);
#12545=ORIENTED_EDGE('',*,*,#9336,.T.);
#12546=ORIENTED_EDGE('',*,*,#9340,.T.);
#12547=ORIENTED_EDGE('',*,*,#9319,.T.);
#12548=ORIENTED_EDGE('',*,*,#9322,.T.);
#12549=ORIENTED_EDGE('',*,*,#9312,.T.);
#12550=ORIENTED_EDGE('',*,*,#9316,.T.);
#12551=ORIENTED_EDGE('',*,*,#9295,.T.);
#12552=ORIENTED_EDGE('',*,*,#9298,.T.);
#12553=ORIENTED_EDGE('',*,*,#9288,.T.);
#12554=ORIENTED_EDGE('',*,*,#9292,.T.);
#12555=ORIENTED_EDGE('',*,*,#9271,.T.);
#12556=ORIENTED_EDGE('',*,*,#9274,.T.);
#12557=ORIENTED_EDGE('',*,*,#9264,.T.);
#12558=ORIENTED_EDGE('',*,*,#9268,.T.);
#12559=ORIENTED_EDGE('',*,*,#9247,.T.);
#12560=ORIENTED_EDGE('',*,*,#9250,.T.);
#12561=ORIENTED_EDGE('',*,*,#9240,.T.);
#12562=ORIENTED_EDGE('',*,*,#9244,.T.);
#12563=ORIENTED_EDGE('',*,*,#9223,.T.);
#12564=ORIENTED_EDGE('',*,*,#9226,.T.);
#12565=ORIENTED_EDGE('',*,*,#9216,.T.);
#12566=ORIENTED_EDGE('',*,*,#9220,.T.);
#12567=ORIENTED_EDGE('',*,*,#9530,.T.);
#12568=ORIENTED_EDGE('',*,*,#9533,.T.);
#12569=ORIENTED_EDGE('',*,*,#9535,.T.);
#12570=ORIENTED_EDGE('',*,*,#9536,.F.);
#15279=CYLINDRICAL_SURFACE('',#17891,0.225000000000001);
#15280=CYLINDRICAL_SURFACE('',#17894,0.225000000000001);
#15281=CYLINDRICAL_SURFACE('',#17897,1.525);
#15282=CYLINDRICAL_SURFACE('',#17911,4.);
#15686=ADVANCED_FACE('',(#2376),#1726,.F.);
#15687=ADVANCED_FACE('',(#2377),#1727,.F.);
#15688=ADVANCED_FACE('',(#2378),#1728,.F.);
#15689=ADVANCED_FACE('',(#2379),#1729,.F.);
#15690=ADVANCED_FACE('',(#2380),#1730,.T.);
#15691=ADVANCED_FACE('',(#2381),#1731,.F.);
#15692=ADVANCED_FACE('',(#2382),#1732,.F.);
#15693=ADVANCED_FACE('',(#2383),#1733,.F.);
#15694=ADVANCED_FACE('',(#2384),#1734,.F.);
#15695=ADVANCED_FACE('',(#2385),#1735,.T.);
#15696=ADVANCED_FACE('',(#2386),#1736,.F.);
#15697=ADVANCED_FACE('',(#2387),#1737,.F.);
#15698=ADVANCED_FACE('',(#2388),#1738,.F.);
#15699=ADVANCED_FACE('',(#2389),#1739,.F.);
#15700=ADVANCED_FACE('',(#2390),#1740,.T.);
#15701=ADVANCED_FACE('',(#2391),#1741,.F.);
#15702=ADVANCED_FACE('',(#2392),#1742,.F.);
#15703=ADVANCED_FACE('',(#2393),#1743,.F.);
#15704=ADVANCED_FACE('',(#2394),#1744,.F.);
#15705=ADVANCED_FACE('',(#2395),#1745,.T.);
#15706=ADVANCED_FACE('',(#2396),#1746,.F.);
#15707=ADVANCED_FACE('',(#2397),#1747,.F.);
#15708=ADVANCED_FACE('',(#2398),#1748,.F.);
#15709=ADVANCED_FACE('',(#2399),#1749,.F.);
#15710=ADVANCED_FACE('',(#2400),#1750,.T.);
#15711=ADVANCED_FACE('',(#2401),#1751,.F.);
#15712=ADVANCED_FACE('',(#2402),#1752,.F.);
#15713=ADVANCED_FACE('',(#2403),#1753,.F.);
#15714=ADVANCED_FACE('',(#2404),#1754,.F.);
#15715=ADVANCED_FACE('',(#2405),#1755,.T.);
#15716=ADVANCED_FACE('',(#2406),#1756,.F.);
#15717=ADVANCED_FACE('',(#2407),#1757,.F.);
#15718=ADVANCED_FACE('',(#2408),#1758,.F.);
#15719=ADVANCED_FACE('',(#2409),#1759,.F.);
#15720=ADVANCED_FACE('',(#2410),#1760,.T.);
#15721=ADVANCED_FACE('',(#2411),#1761,.F.);
#15722=ADVANCED_FACE('',(#2412),#1762,.F.);
#15723=ADVANCED_FACE('',(#2413),#1763,.F.);
#15724=ADVANCED_FACE('',(#2414),#1764,.F.);
#15725=ADVANCED_FACE('',(#2415),#1765,.T.);
#15726=ADVANCED_FACE('',(#2416),#1766,.F.);
#15727=ADVANCED_FACE('',(#2417),#1767,.F.);
#15728=ADVANCED_FACE('',(#2418),#1768,.F.);
#15729=ADVANCED_FACE('',(#2419),#1769,.F.);
#15730=ADVANCED_FACE('',(#2420),#1770,.T.);
#15731=ADVANCED_FACE('',(#2421),#1771,.F.);
#15732=ADVANCED_FACE('',(#2422),#1772,.F.);
#15733=ADVANCED_FACE('',(#2423),#1773,.F.);
#15734=ADVANCED_FACE('',(#2424),#1774,.F.);
#15735=ADVANCED_FACE('',(#2425),#1775,.T.);
#15736=ADVANCED_FACE('',(#2426),#1776,.F.);
#15737=ADVANCED_FACE('',(#2427),#1777,.F.);
#15738=ADVANCED_FACE('',(#2428),#1778,.F.);
#15739=ADVANCED_FACE('',(#2429),#1779,.F.);
#15740=ADVANCED_FACE('',(#2430),#1780,.T.);
#15741=ADVANCED_FACE('',(#2431),#1781,.F.);
#15742=ADVANCED_FACE('',(#2432),#1782,.F.);
#15743=ADVANCED_FACE('',(#2433),#1783,.F.);
#15744=ADVANCED_FACE('',(#2434),#1784,.F.);
#15745=ADVANCED_FACE('',(#2435),#1785,.T.);
#15746=ADVANCED_FACE('',(#2436),#1786,.F.);
#15747=ADVANCED_FACE('',(#2437),#1787,.F.);
#15748=ADVANCED_FACE('',(#2438),#1788,.F.);
#15749=ADVANCED_FACE('',(#2439),#1789,.F.);
#15750=ADVANCED_FACE('',(#2440),#1790,.T.);
#15751=ADVANCED_FACE('',(#2441),#1791,.F.);
#15752=ADVANCED_FACE('',(#2442),#1792,.F.);
#15753=ADVANCED_FACE('',(#2443),#1793,.F.);
#15754=ADVANCED_FACE('',(#2444),#1794,.F.);
#15755=ADVANCED_FACE('',(#2445),#1795,.T.);
#15756=ADVANCED_FACE('',(#2446),#1796,.F.);
#15757=ADVANCED_FACE('',(#2447),#1797,.F.);
#15758=ADVANCED_FACE('',(#2448),#1798,.F.);
#15759=ADVANCED_FACE('',(#2449),#1799,.F.);
#15760=ADVANCED_FACE('',(#2450),#1800,.T.);
#15761=ADVANCED_FACE('',(#2451),#1801,.F.);
#15762=ADVANCED_FACE('',(#2452),#1802,.F.);
#15763=ADVANCED_FACE('',(#2453),#1803,.F.);
#15764=ADVANCED_FACE('',(#2454),#1804,.F.);
#15765=ADVANCED_FACE('',(#2455),#1805,.T.);
#15766=ADVANCED_FACE('',(#2456),#1806,.F.);
#15767=ADVANCED_FACE('',(#2457),#1807,.F.);
#15768=ADVANCED_FACE('',(#2458),#1808,.F.);
#15769=ADVANCED_FACE('',(#2459),#1809,.F.);
#15770=ADVANCED_FACE('',(#2460),#1810,.T.);
#15771=ADVANCED_FACE('',(#2461),#1811,.F.);
#15772=ADVANCED_FACE('',(#2462),#1812,.F.);
#15773=ADVANCED_FACE('',(#2463),#1813,.F.);
#15774=ADVANCED_FACE('',(#2464),#1814,.F.);
#15775=ADVANCED_FACE('',(#2465),#1815,.T.);
#15776=ADVANCED_FACE('',(#2466),#1816,.F.);
#15777=ADVANCED_FACE('',(#2467),#1817,.F.);
#15778=ADVANCED_FACE('',(#2468),#1818,.F.);
#15779=ADVANCED_FACE('',(#2469),#1819,.F.);
#15780=ADVANCED_FACE('',(#2470),#1820,.T.);
#15781=ADVANCED_FACE('',(#2471),#1821,.F.);
#15782=ADVANCED_FACE('',(#2472),#1822,.F.);
#15783=ADVANCED_FACE('',(#2473),#1823,.F.);
#15784=ADVANCED_FACE('',(#2474),#1824,.F.);
#15785=ADVANCED_FACE('',(#2475),#1825,.T.);
#15786=ADVANCED_FACE('',(#2476),#1826,.F.);
#15787=ADVANCED_FACE('',(#2477),#1827,.F.);
#15788=ADVANCED_FACE('',(#2478),#1828,.F.);
#15789=ADVANCED_FACE('',(#2479),#1829,.F.);
#15790=ADVANCED_FACE('',(#2480),#1830,.T.);
#15791=ADVANCED_FACE('',(#2481),#1831,.F.);
#15792=ADVANCED_FACE('',(#2482),#1832,.F.);
#15793=ADVANCED_FACE('',(#2483),#1833,.F.);
#15794=ADVANCED_FACE('',(#2484),#1834,.F.);
#15795=ADVANCED_FACE('',(#2485),#1835,.T.);
#15796=ADVANCED_FACE('',(#2486),#1836,.F.);
#15797=ADVANCED_FACE('',(#2487),#1837,.F.);
#15798=ADVANCED_FACE('',(#2488),#1838,.F.);
#15799=ADVANCED_FACE('',(#2489),#1839,.F.);
#15800=ADVANCED_FACE('',(#2490),#1840,.T.);
#15801=ADVANCED_FACE('',(#2491),#1841,.F.);
#15802=ADVANCED_FACE('',(#2492),#1842,.F.);
#15803=ADVANCED_FACE('',(#2493),#1843,.F.);
#15804=ADVANCED_FACE('',(#2494),#1844,.F.);
#15805=ADVANCED_FACE('',(#2495),#1845,.T.);
#15806=ADVANCED_FACE('',(#2496),#15279,.F.);
#15807=ADVANCED_FACE('',(#2497),#15280,.F.);
#15808=ADVANCED_FACE('',(#2498),#15281,.F.);
#15809=ADVANCED_FACE('',(#2499),#1846,.T.);
#15810=ADVANCED_FACE('',(#2500),#1847,.T.);
#15811=ADVANCED_FACE('',(#2501),#1848,.T.);
#15812=ADVANCED_FACE('',(#2502),#1849,.T.);
#15813=ADVANCED_FACE('',(#2503),#1850,.T.);
#15814=ADVANCED_FACE('',(#2504),#1851,.T.);
#15815=ADVANCED_FACE('',(#2505,#1506,#1507,#1508),#1852,.F.);
#15816=ADVANCED_FACE('',(#2506),#1853,.T.);
#15817=ADVANCED_FACE('',(#2507,#1509,#1510,#1511,#1512,#1513,#1514,#1515,
#1516,#1517,#1518,#1519,#1520,#1521,#1522,#1523,#1524,#1525,#1526,#1527,
#1528,#1529,#1530,#1531,#1532,#1533,#1534,#1535),#1854,.T.);
#15818=ADVANCED_FACE('',(#2508),#15282,.T.);
#16408=CLOSED_SHELL('',(#15686,#15687,#15688,#15689,#15690,#15691,#15692,
#15693,#15694,#15695,#15696,#15697,#15698,#15699,#15700,#15701,#15702,#15703,
#15704,#15705,#15706,#15707,#15708,#15709,#15710,#15711,#15712,#15713,#15714,
#15715,#15716,#15717,#15718,#15719,#15720,#15721,#15722,#15723,#15724,#15725,
#15726,#15727,#15728,#15729,#15730,#15731,#15732,#15733,#15734,#15735,#15736,
#15737,#15738,#15739,#15740,#15741,#15742,#15743,#15744,#15745,#15746,#15747,
#15748,#15749,#15750,#15751,#15752,#15753,#15754,#15755,#15756,#15757,#15758,
#15759,#15760,#15761,#15762,#15763,#15764,#15765,#15766,#15767,#15768,#15769,
#15770,#15771,#15772,#15773,#15774,#15775,#15776,#15777,#15778,#15779,#15780,
#15781,#15782,#15783,#15784,#15785,#15786,#15787,#15788,#15789,#15790,#15791,
#15792,#15793,#15794,#15795,#15796,#15797,#15798,#15799,#15800,#15801,#15802,
#15803,#15804,#15805,#15806,#15807,#15808,#15809,#15810,#15811,#15812,#15813,
#15814,#15815,#15816,#15817,#15818));
#17770=AXIS2_PLACEMENT_3D('',#25157,#20247,#20248);
#17771=AXIS2_PLACEMENT_3D('',#25158,#20249,#20250);
#17772=AXIS2_PLACEMENT_3D('',#25167,#20255,#20256);
#17773=AXIS2_PLACEMENT_3D('',#25173,#20260,#20261);
#17774=AXIS2_PLACEMENT_3D('',#25179,#20265,#20266);
#17775=AXIS2_PLACEMENT_3D('',#25182,#20269,#20270);
#17776=AXIS2_PLACEMENT_3D('',#25183,#20271,#20272);
#17777=AXIS2_PLACEMENT_3D('',#25192,#20277,#20278);
#17778=AXIS2_PLACEMENT_3D('',#25198,#20282,#20283);
#17779=AXIS2_PLACEMENT_3D('',#25204,#20287,#20288);
#17780=AXIS2_PLACEMENT_3D('',#25207,#20291,#20292);
#17781=AXIS2_PLACEMENT_3D('',#25208,#20293,#20294);
#17782=AXIS2_PLACEMENT_3D('',#25217,#20299,#20300);
#17783=AXIS2_PLACEMENT_3D('',#25223,#20304,#20305);
#17784=AXIS2_PLACEMENT_3D('',#25229,#20309,#20310);
#17785=AXIS2_PLACEMENT_3D('',#25232,#20313,#20314);
#17786=AXIS2_PLACEMENT_3D('',#25233,#20315,#20316);
#17787=AXIS2_PLACEMENT_3D('',#25242,#20321,#20322);
#17788=AXIS2_PLACEMENT_3D('',#25248,#20326,#20327);
#17789=AXIS2_PLACEMENT_3D('',#25254,#20331,#20332);
#17790=AXIS2_PLACEMENT_3D('',#25257,#20335,#20336);
#17791=AXIS2_PLACEMENT_3D('',#25258,#20337,#20338);
#17792=AXIS2_PLACEMENT_3D('',#25267,#20343,#20344);
#17793=AXIS2_PLACEMENT_3D('',#25273,#20348,#20349);
#17794=AXIS2_PLACEMENT_3D('',#25279,#20353,#20354);
#17795=AXIS2_PLACEMENT_3D('',#25282,#20357,#20358);
#17796=AXIS2_PLACEMENT_3D('',#25283,#20359,#20360);
#17797=AXIS2_PLACEMENT_3D('',#25292,#20365,#20366);
#17798=AXIS2_PLACEMENT_3D('',#25298,#20370,#20371);
#17799=AXIS2_PLACEMENT_3D('',#25304,#20375,#20376);
#17800=AXIS2_PLACEMENT_3D('',#25307,#20379,#20380);
#17801=AXIS2_PLACEMENT_3D('',#25308,#20381,#20382);
#17802=AXIS2_PLACEMENT_3D('',#25317,#20387,#20388);
#17803=AXIS2_PLACEMENT_3D('',#25323,#20392,#20393);
#17804=AXIS2_PLACEMENT_3D('',#25329,#20397,#20398);
#17805=AXIS2_PLACEMENT_3D('',#25332,#20401,#20402);
#17806=AXIS2_PLACEMENT_3D('',#25333,#20403,#20404);
#17807=AXIS2_PLACEMENT_3D('',#25342,#20409,#20410);
#17808=AXIS2_PLACEMENT_3D('',#25348,#20414,#20415);
#17809=AXIS2_PLACEMENT_3D('',#25354,#20419,#20420);
#17810=AXIS2_PLACEMENT_3D('',#25357,#20423,#20424);
#17811=AXIS2_PLACEMENT_3D('',#25358,#20425,#20426);
#17812=AXIS2_PLACEMENT_3D('',#25367,#20431,#20432);
#17813=AXIS2_PLACEMENT_3D('',#25373,#20436,#20437);
#17814=AXIS2_PLACEMENT_3D('',#25379,#20441,#20442);
#17815=AXIS2_PLACEMENT_3D('',#25382,#20445,#20446);
#17816=AXIS2_PLACEMENT_3D('',#25383,#20447,#20448);
#17817=AXIS2_PLACEMENT_3D('',#25392,#20453,#20454);
#17818=AXIS2_PLACEMENT_3D('',#25398,#20458,#20459);
#17819=AXIS2_PLACEMENT_3D('',#25404,#20463,#20464);
#17820=AXIS2_PLACEMENT_3D('',#25407,#20467,#20468);
#17821=AXIS2_PLACEMENT_3D('',#25408,#20469,#20470);
#17822=AXIS2_PLACEMENT_3D('',#25417,#20475,#20476);
#17823=AXIS2_PLACEMENT_3D('',#25423,#20480,#20481);
#17824=AXIS2_PLACEMENT_3D('',#25429,#20485,#20486);
#17825=AXIS2_PLACEMENT_3D('',#25432,#20489,#20490);
#17826=AXIS2_PLACEMENT_3D('',#25433,#20491,#20492);
#17827=AXIS2_PLACEMENT_3D('',#25442,#20497,#20498);
#17828=AXIS2_PLACEMENT_3D('',#25448,#20502,#20503);
#17829=AXIS2_PLACEMENT_3D('',#25454,#20507,#20508);
#17830=AXIS2_PLACEMENT_3D('',#25457,#20511,#20512);
#17831=AXIS2_PLACEMENT_3D('',#25458,#20513,#20514);
#17832=AXIS2_PLACEMENT_3D('',#25467,#20519,#20520);
#17833=AXIS2_PLACEMENT_3D('',#25473,#20524,#20525);
#17834=AXIS2_PLACEMENT_3D('',#25479,#20529,#20530);
#17835=AXIS2_PLACEMENT_3D('',#25482,#20533,#20534);
#17836=AXIS2_PLACEMENT_3D('',#25483,#20535,#20536);
#17837=AXIS2_PLACEMENT_3D('',#25492,#20541,#20542);
#17838=AXIS2_PLACEMENT_3D('',#25498,#20546,#20547);
#17839=AXIS2_PLACEMENT_3D('',#25504,#20551,#20552);
#17840=AXIS2_PLACEMENT_3D('',#25507,#20555,#20556);
#17841=AXIS2_PLACEMENT_3D('',#25508,#20557,#20558);
#17842=AXIS2_PLACEMENT_3D('',#25517,#20563,#20564);
#17843=AXIS2_PLACEMENT_3D('',#25523,#20568,#20569);
#17844=AXIS2_PLACEMENT_3D('',#25529,#20573,#20574);
#17845=AXIS2_PLACEMENT_3D('',#25532,#20577,#20578);
#17846=AXIS2_PLACEMENT_3D('',#25533,#20579,#20580);
#17847=AXIS2_PLACEMENT_3D('',#25542,#20585,#20586);
#17848=AXIS2_PLACEMENT_3D('',#25548,#20590,#20591);
#17849=AXIS2_PLACEMENT_3D('',#25554,#20595,#20596);
#17850=AXIS2_PLACEMENT_3D('',#25557,#20599,#20600);
#17851=AXIS2_PLACEMENT_3D('',#25558,#20601,#20602);
#17852=AXIS2_PLACEMENT_3D('',#25567,#20607,#20608);
#17853=AXIS2_PLACEMENT_3D('',#25573,#20612,#20613);
#17854=AXIS2_PLACEMENT_3D('',#25579,#20617,#20618);
#17855=AXIS2_PLACEMENT_3D('',#25582,#20621,#20622);
#17856=AXIS2_PLACEMENT_3D('',#25583,#20623,#20624);
#17857=AXIS2_PLACEMENT_3D('',#25592,#20629,#20630);
#17858=AXIS2_PLACEMENT_3D('',#25598,#20634,#20635);
#17859=AXIS2_PLACEMENT_3D('',#25604,#20639,#20640);
#17860=AXIS2_PLACEMENT_3D('',#25607,#20643,#20644);
#17861=AXIS2_PLACEMENT_3D('',#25608,#20645,#20646);
#17862=AXIS2_PLACEMENT_3D('',#25617,#20651,#20652);
#17863=AXIS2_PLACEMENT_3D('',#25623,#20656,#20657);
#17864=AXIS2_PLACEMENT_3D('',#25629,#20661,#20662);
#17865=AXIS2_PLACEMENT_3D('',#25632,#20665,#20666);
#17866=AXIS2_PLACEMENT_3D('',#25633,#20667,#20668);
#17867=AXIS2_PLACEMENT_3D('',#25642,#20673,#20674);
#17868=AXIS2_PLACEMENT_3D('',#25648,#20678,#20679);
#17869=AXIS2_PLACEMENT_3D('',#25654,#20683,#20684);
#17870=AXIS2_PLACEMENT_3D('',#25657,#20687,#20688);
#17871=AXIS2_PLACEMENT_3D('',#25658,#20689,#20690);
#17872=AXIS2_PLACEMENT_3D('',#25667,#20695,#20696);
#17873=AXIS2_PLACEMENT_3D('',#25673,#20700,#20701);
#17874=AXIS2_PLACEMENT_3D('',#25679,#20705,#20706);
#17875=AXIS2_PLACEMENT_3D('',#25682,#20709,#20710);
#17876=AXIS2_PLACEMENT_3D('',#25683,#20711,#20712);
#17877=AXIS2_PLACEMENT_3D('',#25692,#20717,#20718);
#17878=AXIS2_PLACEMENT_3D('',#25698,#20722,#20723);
#17879=AXIS2_PLACEMENT_3D('',#25704,#20727,#20728);
#17880=AXIS2_PLACEMENT_3D('',#25707,#20731,#20732);
#17881=AXIS2_PLACEMENT_3D('',#25708,#20733,#20734);
#17882=AXIS2_PLACEMENT_3D('',#25717,#20739,#20740);
#17883=AXIS2_PLACEMENT_3D('',#25723,#20744,#20745);
#17884=AXIS2_PLACEMENT_3D('',#25729,#20749,#20750);
#17885=AXIS2_PLACEMENT_3D('',#25732,#20753,#20754);
#17886=AXIS2_PLACEMENT_3D('',#25733,#20755,#20756);
#17887=AXIS2_PLACEMENT_3D('',#25742,#20761,#20762);
#17888=AXIS2_PLACEMENT_3D('',#25748,#20766,#20767);
#17889=AXIS2_PLACEMENT_3D('',#25754,#20771,#20772);
#17890=AXIS2_PLACEMENT_3D('',#25757,#20775,#20776);
#17891=AXIS2_PLACEMENT_3D('',#25758,#20777,#20778);
#17892=AXIS2_PLACEMENT_3D('',#25760,#20779,#20780);
#17893=AXIS2_PLACEMENT_3D('',#25763,#20782,#20783);
#17894=AXIS2_PLACEMENT_3D('',#25764,#20784,#20785);
#17895=AXIS2_PLACEMENT_3D('',#25766,#20786,#20787);
#17896=AXIS2_PLACEMENT_3D('',#25769,#20789,#20790);
#17897=AXIS2_PLACEMENT_3D('',#25770,#20791,#20792);
#17898=AXIS2_PLACEMENT_3D('',#25772,#20793,#20794);
#17899=AXIS2_PLACEMENT_3D('',#25775,#20796,#20797);
#17900=AXIS2_PLACEMENT_3D('',#25776,#20798,#20799);
#17901=AXIS2_PLACEMENT_3D('',#25785,#20804,#20805);
#17902=AXIS2_PLACEMENT_3D('',#25794,#20810,#20811);
#17903=AXIS2_PLACEMENT_3D('',#25800,#20815,#20816);
#17904=AXIS2_PLACEMENT_3D('',#25806,#20820,#20821);
#17905=AXIS2_PLACEMENT_3D('',#25809,#20824,#20825);
#17906=AXIS2_PLACEMENT_3D('',#25815,#20829,#20830);
#17907=AXIS2_PLACEMENT_3D('',#25818,#20832,#20833);
#17908=AXIS2_PLACEMENT_3D('',#25819,#20834,#20835);
#17909=AXIS2_PLACEMENT_3D('',#25823,#20838,#20839);
#17910=AXIS2_PLACEMENT_3D('',#25824,#20840,#20841);
#17911=AXIS2_PLACEMENT_3D('',#25825,#20842,#20843);
#20247=DIRECTION('axis',(0.,0.,1.));
#20248=DIRECTION('refdir',(1.,0.,0.));
#20249=DIRECTION('center_axis',(0.96592582628908,0.,-0.258819045102476));
#20250=DIRECTION('ref_axis',(-0.258819045102476,0.,-0.96592582628908));
#20251=DIRECTION('',(0.258819045102476,0.,0.96592582628908));
#20252=DIRECTION('',(0.,1.,0.));
#20253=DIRECTION('',(0.258819045102476,0.,0.96592582628908));
#20254=DIRECTION('',(0.,1.,0.));
#20255=DIRECTION('center_axis',(0.25108343875234,0.,0.967965447102478));
#20256=DIRECTION('ref_axis',(0.967965447102478,0.,-0.25108343875234));
#20257=DIRECTION('',(-0.967965447102478,0.,0.25108343875234));
#20258=DIRECTION('',(-0.967965447102478,0.,0.25108343875234));
#20259=DIRECTION('',(0.,1.,0.));
#20260=DIRECTION('center_axis',(-0.965925826289075,0.,0.258819045102495));
#20261=DIRECTION('ref_axis',(0.258819045102495,0.,0.965925826289075));
#20262=DIRECTION('',(-0.258819045102495,0.,-0.965925826289075));
#20263=DIRECTION('',(-0.258819045102495,0.,-0.965925826289075));
#20264=DIRECTION('',(0.,1.,0.));
#20265=DIRECTION('center_axis',(-0.266538087122156,0.,-0.963824386552479));
#20266=DIRECTION('ref_axis',(-0.963824386552479,0.,0.266538087122156));
#20267=DIRECTION('',(0.963824386552479,0.,-0.266538087122156));
#20268=DIRECTION('',(0.963824386552479,0.,-0.266538087122156));
#20269=DIRECTION('center_axis',(0.,1.,0.));
#20270=DIRECTION('ref_axis',(1.,0.,0.));
#20271=DIRECTION('center_axis',(0.866025403784429,0.,-0.500000000000017));
#20272=DIRECTION('ref_axis',(-0.500000000000017,0.,-0.866025403784429));
#20273=DIRECTION('',(0.500000000000017,0.,0.866025403784429));
#20274=DIRECTION('',(0.,1.,0.));
#20275=DIRECTION('',(0.500000000000017,0.,0.866025403784429));
#20276=DIRECTION('',(0.,1.,0.));
#20277=DIRECTION('center_axis',(0.493055870755657,0.,0.869997648452788));
#20278=DIRECTION('ref_axis',(0.869997648452788,0.,-0.493055870755657));
#20279=DIRECTION('',(-0.869997648452788,0.,0.493055870755657));
#20280=DIRECTION('',(-0.869997648452788,0.,0.493055870755657));
#20281=DIRECTION('',(0.,1.,0.));
#20282=DIRECTION('center_axis',(-0.866025403784438,0.,0.500000000000001));
#20283=DIRECTION('ref_axis',(0.500000000000001,0.,0.866025403784438));
#20284=DIRECTION('',(-0.500000000000001,0.,-0.866025403784438));
#20285=DIRECTION('',(-0.500000000000001,0.,-0.866025403784438));
#20286=DIRECTION('',(0.,1.,0.));
#20287=DIRECTION('center_axis',(-0.506912129415013,0.,-0.861997733785848));
#20288=DIRECTION('ref_axis',(-0.861997733785848,0.,0.506912129415013));
#20289=DIRECTION('',(0.861997733785848,0.,-0.506912129415013));
#20290=DIRECTION('',(0.861997733785848,0.,-0.506912129415013));
#20291=DIRECTION('center_axis',(0.,1.,0.));
#20292=DIRECTION('ref_axis',(1.,0.,0.));
#20293=DIRECTION('center_axis',(0.70710678118654,0.,-0.707106781186555));
#20294=DIRECTION('ref_axis',(-0.707106781186555,0.,-0.70710678118654));
#20295=DIRECTION('',(0.707106781186555,0.,0.70710678118654));
#20296=DIRECTION('',(0.,1.,0.));
#20297=DIRECTION('',(0.707106781186555,0.,0.70710678118654));
#20298=DIRECTION('',(0.,1.,0.));
#20299=DIRECTION('center_axis',(0.70142735998032,0.,0.712740947800137));
#20300=DIRECTION('ref_axis',(0.712740947800137,0.,-0.70142735998032));
#20301=DIRECTION('',(-0.712740947800137,0.,0.70142735998032));
#20302=DIRECTION('',(-0.712740947800137,0.,0.70142735998032));
#20303=DIRECTION('',(0.,1.,0.));
#20304=DIRECTION('center_axis',(-0.707106781186564,0.,0.707106781186531));
#20305=DIRECTION('ref_axis',(0.707106781186531,0.,0.707106781186564));
#20306=DIRECTION('',(-0.707106781186531,0.,-0.707106781186564));
#20307=DIRECTION('',(-0.707106781186531,0.,-0.707106781186564));
#20308=DIRECTION('',(0.,1.,0.));
#20309=DIRECTION('center_axis',(-0.712740947800136,0.,-0.701427359980322));
#20310=DIRECTION('ref_axis',(-0.701427359980322,0.,0.712740947800136));
#20311=DIRECTION('',(0.701427359980322,0.,-0.712740947800136));
#20312=DIRECTION('',(0.701427359980322,0.,-0.712740947800136));
#20313=DIRECTION('center_axis',(0.,1.,0.));
#20314=DIRECTION('ref_axis',(1.,0.,0.));
#20315=DIRECTION('center_axis',(0.500000000000008,0.,-0.866025403784434));
#20316=DIRECTION('ref_axis',(-0.866025403784434,0.,-0.500000000000008));
#20317=DIRECTION('',(0.866025403784434,0.,0.500000000000008));
#20318=DIRECTION('',(0.,1.,0.));
#20319=DIRECTION('',(0.866025403784434,0.,0.500000000000008));
#20320=DIRECTION('',(0.,1.,0.));
#20321=DIRECTION('center_axis',(0.861997733785848,0.,0.506912129415013));
#20322=DIRECTION('ref_axis',(0.506912129415013,0.,-0.861997733785848));
#20323=DIRECTION('',(-0.506912129415013,0.,0.861997733785848));
#20324=DIRECTION('',(-0.506912129415013,0.,0.861997733785848));
#20325=DIRECTION('',(0.,1.,0.));
#20326=DIRECTION('center_axis',(-0.500000000000017,0.,0.866025403784429));
#20327=DIRECTION('ref_axis',(0.866025403784429,0.,0.500000000000017));
#20328=DIRECTION('',(-0.866025403784429,0.,-0.500000000000017));
#20329=DIRECTION('',(-0.866025403784429,0.,-0.500000000000017));
#20330=DIRECTION('',(0.,1.,0.));
#20331=DIRECTION('center_axis',(-0.869997648452789,0.,-0.493055870755654));
#20332=DIRECTION('ref_axis',(-0.493055870755654,0.,0.869997648452789));
#20333=DIRECTION('',(0.493055870755654,0.,-0.869997648452789));
#20334=DIRECTION('',(0.493055870755654,0.,-0.869997648452789));
#20335=DIRECTION('center_axis',(0.,1.,0.));
#20336=DIRECTION('ref_axis',(1.,0.,0.));
#20337=DIRECTION('center_axis',(0.258819045102528,0.,-0.965925826289066));
#20338=DIRECTION('ref_axis',(-0.965925826289066,0.,-0.258819045102528));
#20339=DIRECTION('',(0.965925826289066,0.,0.258819045102528));
#20340=DIRECTION('',(0.,1.,0.));
#20341=DIRECTION('',(0.965925826289066,0.,0.258819045102528));
#20342=DIRECTION('',(0.,1.,0.));
#20343=DIRECTION('center_axis',(0.96382438655248,0.,0.26653808712215));
#20344=DIRECTION('ref_axis',(0.26653808712215,0.,-0.96382438655248));
#20345=DIRECTION('',(-0.26653808712215,0.,0.96382438655248));
#20346=DIRECTION('',(-0.26653808712215,0.,0.96382438655248));
#20347=DIRECTION('',(0.,1.,0.));
#20348=DIRECTION('center_axis',(-0.258819045102533,0.,0.965925826289065));
#20349=DIRECTION('ref_axis',(0.965925826289065,0.,0.258819045102533));
#20350=DIRECTION('',(-0.965925826289065,0.,-0.258819045102533));
#20351=DIRECTION('',(-0.965925826289065,0.,-0.258819045102533));
#20352=DIRECTION('',(0.,1.,0.));
#20353=DIRECTION('center_axis',(-0.967965447102477,0.,-0.251083438752344));
#20354=DIRECTION('ref_axis',(-0.251083438752344,0.,0.967965447102477));
#20355=DIRECTION('',(0.251083438752344,0.,-0.967965447102477));
#20356=DIRECTION('',(0.251083438752344,0.,-0.967965447102477));
#20357=DIRECTION('center_axis',(0.,1.,0.));
#20358=DIRECTION('ref_axis',(1.,0.,0.));
#20359=DIRECTION('center_axis',(0.,0.,-1.));
#20360=DIRECTION('ref_axis',(-1.,0.,0.));
#20361=DIRECTION('',(1.,0.,0.));
#20362=DIRECTION('',(0.,1.,0.));
#20363=DIRECTION('',(1.,0.,0.));
#20364=DIRECTION('',(0.,1.,0.));
#20365=DIRECTION('center_axis',(0.999968000170666,0.,0.00799991466693405));
#20366=DIRECTION('ref_axis',(0.00799991466693405,0.,-0.999968000170666));
#20367=DIRECTION('',(-0.00799991466693405,0.,0.999968000170666));
#20368=DIRECTION('',(-0.00799991466693405,0.,0.999968000170666));
#20369=DIRECTION('',(0.,1.,0.));
#20370=DIRECTION('center_axis',(0.,0.,1.));
#20371=DIRECTION('ref_axis',(1.,0.,0.));
#20372=DIRECTION('',(-1.,0.,0.));
#20373=DIRECTION('',(-1.,0.,0.));
#20374=DIRECTION('',(0.,1.,0.));
#20375=DIRECTION('center_axis',(-0.999968000170666,0.,0.00799991466694293));
#20376=DIRECTION('ref_axis',(0.00799991466694293,0.,0.999968000170666));
#20377=DIRECTION('',(-0.00799991466694293,0.,-0.999968000170666));
#20378=DIRECTION('',(-0.00799991466694293,0.,-0.999968000170666));
#20379=DIRECTION('center_axis',(0.,1.,0.));
#20380=DIRECTION('ref_axis',(1.,0.,0.));
#20381=DIRECTION('center_axis',(-0.258819045102499,0.,-0.965925826289074));
#20382=DIRECTION('ref_axis',(-0.965925826289074,0.,0.258819045102499));
#20383=DIRECTION('',(0.965925826289074,0.,-0.258819045102499));
#20384=DIRECTION('',(0.,1.,0.));
#20385=DIRECTION('',(0.965925826289074,0.,-0.258819045102499));
#20386=DIRECTION('',(0.,1.,0.));
#20387=DIRECTION('center_axis',(0.967965447102479,0.,-0.251083438752336));
#20388=DIRECTION('ref_axis',(-0.251083438752336,0.,-0.967965447102479));
#20389=DIRECTION('',(0.251083438752336,0.,0.967965447102479));
#20390=DIRECTION('',(0.251083438752336,0.,0.967965447102479));
#20391=DIRECTION('',(0.,1.,0.));
#20392=DIRECTION('center_axis',(0.258819045102534,0.,0.965925826289065));
#20393=DIRECTION('ref_axis',(0.965925826289065,0.,-0.258819045102534));
#20394=DIRECTION('',(-0.965925826289065,0.,0.258819045102534));
#20395=DIRECTION('',(-0.965925826289065,0.,0.258819045102534));
#20396=DIRECTION('',(0.,1.,0.));
#20397=DIRECTION('center_axis',(-0.963824386552478,0.,0.266538087122158));
#20398=DIRECTION('ref_axis',(0.266538087122158,0.,0.963824386552478));
#20399=DIRECTION('',(-0.266538087122158,0.,-0.963824386552478));
#20400=DIRECTION('',(-0.266538087122158,0.,-0.963824386552478));
#20401=DIRECTION('center_axis',(0.,1.,0.));
#20402=DIRECTION('ref_axis',(1.,0.,0.));
#20403=DIRECTION('center_axis',(-0.499999999999982,0.,-0.866025403784449));
#20404=DIRECTION('ref_axis',(-0.866025403784449,0.,0.499999999999982));
#20405=DIRECTION('',(0.866025403784449,0.,-0.499999999999982));
#20406=DIRECTION('',(0.,1.,0.));
#20407=DIRECTION('',(0.866025403784449,0.,-0.499999999999982));
#20408=DIRECTION('',(0.,1.,0.));
#20409=DIRECTION('center_axis',(0.869997648452789,0.,-0.493055870755654));
#20410=DIRECTION('ref_axis',(-0.493055870755654,0.,-0.869997648452789));
#20411=DIRECTION('',(0.493055870755654,0.,0.869997648452789));
#20412=DIRECTION('',(0.493055870755654,0.,0.869997648452789));
#20413=DIRECTION('',(0.,1.,0.));
#20414=DIRECTION('center_axis',(0.500000000000001,0.,0.866025403784438));
#20415=DIRECTION('ref_axis',(0.866025403784438,0.,-0.500000000000001));
#20416=DIRECTION('',(-0.866025403784438,0.,0.500000000000001));
#20417=DIRECTION('',(-0.866025403784438,0.,0.500000000000001));
#20418=DIRECTION('',(0.,1.,0.));
#20419=DIRECTION('center_axis',(-0.861997733785848,0.,0.506912129415012));
#20420=DIRECTION('ref_axis',(0.506912129415012,0.,0.861997733785848));
#20421=DIRECTION('',(-0.506912129415012,0.,-0.861997733785848));
#20422=DIRECTION('',(-0.506912129415012,0.,-0.861997733785848));
#20423=DIRECTION('center_axis',(0.,1.,0.));
#20424=DIRECTION('ref_axis',(1.,0.,0.));
#20425=DIRECTION('center_axis',(-0.707106781186555,0.,-0.70710678118654));
#20426=DIRECTION('ref_axis',(-0.70710678118654,0.,0.707106781186555));
#20427=DIRECTION('',(0.70710678118654,0.,-0.707106781186555));
#20428=DIRECTION('',(0.,1.,0.));
#20429=DIRECTION('',(0.70710678118654,0.,-0.707106781186555));
#20430=DIRECTION('',(0.,1.,0.));
#20431=DIRECTION('center_axis',(0.712740947800135,0.,-0.701427359980323));
#20432=DIRECTION('ref_axis',(-0.701427359980323,0.,-0.712740947800135));
#20433=DIRECTION('',(0.701427359980323,0.,0.712740947800135));
#20434=DIRECTION('',(0.701427359980323,0.,0.712740947800135));
#20435=DIRECTION('',(0.,1.,0.));
#20436=DIRECTION('center_axis',(0.707106781186539,0.,0.707106781186556));
#20437=DIRECTION('ref_axis',(0.707106781186556,0.,-0.707106781186539));
#20438=DIRECTION('',(-0.707106781186556,0.,0.707106781186539));
#20439=DIRECTION('',(-0.707106781186556,0.,0.707106781186539));
#20440=DIRECTION('',(0.,1.,0.));
#20441=DIRECTION('center_axis',(-0.701427359980323,0.,0.712740947800135));
#20442=DIRECTION('ref_axis',(0.712740947800135,0.,0.701427359980323));
#20443=DIRECTION('',(-0.712740947800135,0.,-0.701427359980323));
#20444=DIRECTION('',(-0.712740947800135,0.,-0.701427359980323));
#20445=DIRECTION('center_axis',(0.,1.,0.));
#20446=DIRECTION('ref_axis',(1.,0.,0.));
#20447=DIRECTION('center_axis',(-0.866025403784425,0.,-0.500000000000023));
#20448=DIRECTION('ref_axis',(-0.500000000000023,0.,0.866025403784425));
#20449=DIRECTION('',(0.500000000000023,0.,-0.866025403784425));
#20450=DIRECTION('',(0.,1.,0.));
#20451=DIRECTION('',(0.500000000000023,0.,-0.866025403784425));
#20452=DIRECTION('',(0.,1.,0.));
#20453=DIRECTION('center_axis',(0.50691212941501,0.,-0.86199773378585));
#20454=DIRECTION('ref_axis',(-0.86199773378585,0.,-0.50691212941501));
#20455=DIRECTION('',(0.86199773378585,0.,0.50691212941501));
#20456=DIRECTION('',(0.86199773378585,0.,0.50691212941501));
#20457=DIRECTION('',(0.,1.,0.));
#20458=DIRECTION('center_axis',(0.866025403784448,0.,0.499999999999983));
#20459=DIRECTION('ref_axis',(0.499999999999983,0.,-0.866025403784448));
#20460=DIRECTION('',(-0.499999999999983,0.,0.866025403784448));
#20461=DIRECTION('',(-0.499999999999983,0.,0.866025403784448));
#20462=DIRECTION('',(0.,1.,0.));
#20463=DIRECTION('center_axis',(-0.493055870755651,0.,0.869997648452791));
#20464=DIRECTION('ref_axis',(0.869997648452791,0.,0.493055870755651));
#20465=DIRECTION('',(-0.869997648452791,0.,-0.493055870755651));
#20466=DIRECTION('',(-0.869997648452791,0.,-0.493055870755651));
#20467=DIRECTION('center_axis',(0.,1.,0.));
#20468=DIRECTION('ref_axis',(1.,0.,0.));
#20469=DIRECTION('center_axis',(-0.965925826289073,0.,-0.258819045102503));
#20470=DIRECTION('ref_axis',(-0.258819045102503,0.,0.965925826289073));
#20471=DIRECTION('',(0.258819045102503,0.,-0.965925826289073));
#20472=DIRECTION('',(0.,1.,0.));
#20473=DIRECTION('',(0.258819045102503,0.,-0.965925826289073));
#20474=DIRECTION('',(0.,1.,0.));
#20475=DIRECTION('center_axis',(0.266538087122153,0.,-0.96382438655248));
#20476=DIRECTION('ref_axis',(-0.96382438655248,0.,-0.266538087122153));
#20477=DIRECTION('',(0.96382438655248,0.,0.266538087122153));
#20478=DIRECTION('',(0.96382438655248,0.,0.266538087122153));
#20479=DIRECTION('',(0.,1.,0.));
#20480=DIRECTION('center_axis',(0.965925826289077,0.,0.258819045102487));
#20481=DIRECTION('ref_axis',(0.258819045102487,0.,-0.965925826289077));
#20482=DIRECTION('',(-0.258819045102487,0.,0.965925826289077));
#20483=DIRECTION('',(-0.258819045102487,0.,0.965925826289077));
#20484=DIRECTION('',(0.,1.,0.));
#20485=DIRECTION('center_axis',(-0.25108343875234,0.,0.967965447102478));
#20486=DIRECTION('ref_axis',(0.967965447102478,0.,0.25108343875234));
#20487=DIRECTION('',(-0.967965447102478,0.,-0.25108343875234));
#20488=DIRECTION('',(-0.967965447102478,0.,-0.25108343875234));
#20489=DIRECTION('center_axis',(0.,1.,0.));
#20490=DIRECTION('ref_axis',(1.,0.,0.));
#20491=DIRECTION('center_axis',(-1.,0.,0.));
#20492=DIRECTION('ref_axis',(0.,0.,1.));
#20493=DIRECTION('',(0.,0.,-1.));
#20494=DIRECTION('',(0.,1.,0.));
#20495=DIRECTION('',(0.,0.,-1.));
#20496=DIRECTION('',(0.,1.,0.));
#20497=DIRECTION('center_axis',(0.00799991466693849,0.,-0.999968000170666));
#20498=DIRECTION('ref_axis',(-0.999968000170666,0.,-0.00799991466693849));
#20499=DIRECTION('',(0.999968000170666,0.,0.00799991466693849));
#20500=DIRECTION('',(0.999968000170666,0.,0.00799991466693849));
#20501=DIRECTION('',(0.,1.,0.));
#20502=DIRECTION('center_axis',(1.,0.,0.));
#20503=DIRECTION('ref_axis',(0.,0.,-1.));
#20504=DIRECTION('',(0.,0.,1.));
#20505=DIRECTION('',(0.,0.,1.));
#20506=DIRECTION('',(0.,1.,0.));
#20507=DIRECTION('center_axis',(0.00799991466693849,0.,0.999968000170666));
#20508=DIRECTION('ref_axis',(0.999968000170666,0.,-0.00799991466693849));
#20509=DIRECTION('',(-0.999968000170666,0.,0.00799991466693849));
#20510=DIRECTION('',(-0.999968000170666,0.,0.00799991466693849));
#20511=DIRECTION('center_axis',(0.,1.,0.));
#20512=DIRECTION('ref_axis',(1.,0.,0.));
#20513=DIRECTION('center_axis',(-0.965925826289065,0.,0.258819045102534));
#20514=DIRECTION('ref_axis',(0.258819045102534,0.,0.965925826289065));
#20515=DIRECTION('',(-0.258819045102534,0.,-0.965925826289065));
#20516=DIRECTION('',(0.,1.,0.));
#20517=DIRECTION('',(-0.258819045102534,0.,-0.965925826289065));
#20518=DIRECTION('',(0.,1.,0.));
#20519=DIRECTION('center_axis',(-0.251083438752344,0.,-0.967965447102477));
#20520=DIRECTION('ref_axis',(-0.967965447102477,0.,0.251083438752344));
#20521=DIRECTION('',(0.967965447102477,0.,-0.251083438752344));
#20522=DIRECTION('',(0.967965447102477,0.,-0.251083438752344));
#20523=DIRECTION('',(0.,1.,0.));
#20524=DIRECTION('center_axis',(0.965925826289061,0.,-0.258819045102548));
#20525=DIRECTION('ref_axis',(-0.258819045102548,0.,-0.965925826289061));
#20526=DIRECTION('',(0.258819045102548,0.,0.965925826289061));
#20527=DIRECTION('',(0.258819045102548,0.,0.965925826289061));
#20528=DIRECTION('',(0.,1.,0.));
#20529=DIRECTION('center_axis',(0.266538087122154,0.,0.963824386552479));
#20530=DIRECTION('ref_axis',(0.963824386552479,0.,-0.266538087122154));
#20531=DIRECTION('',(-0.963824386552479,0.,0.266538087122154));
#20532=DIRECTION('',(-0.963824386552479,0.,0.266538087122154));
#20533=DIRECTION('center_axis',(0.,1.,0.));
#20534=DIRECTION('ref_axis',(1.,0.,0.));
#20535=DIRECTION('center_axis',(-0.866025403784429,0.,0.500000000000017));
#20536=DIRECTION('ref_axis',(0.500000000000017,0.,0.866025403784429));
#20537=DIRECTION('',(-0.500000000000017,0.,-0.866025403784429));
#20538=DIRECTION('',(0.,1.,0.));
#20539=DIRECTION('',(-0.500000000000017,0.,-0.866025403784429));
#20540=DIRECTION('',(0.,1.,0.));
#20541=DIRECTION('center_axis',(-0.493055870755655,0.,-0.869997648452789));
#20542=DIRECTION('ref_axis',(-0.869997648452789,0.,0.493055870755655));
#20543=DIRECTION('',(0.869997648452789,0.,-0.493055870755655));
#20544=DIRECTION('',(0.869997648452789,0.,-0.493055870755655));
#20545=DIRECTION('',(0.,1.,0.));
#20546=DIRECTION('center_axis',(0.866025403784452,0.,-0.499999999999976));
#20547=DIRECTION('ref_axis',(-0.499999999999976,0.,-0.866025403784452));
#20548=DIRECTION('',(0.499999999999976,0.,0.866025403784452));
#20549=DIRECTION('',(0.499999999999976,0.,0.866025403784452));
#20550=DIRECTION('',(0.,1.,0.));
#20551=DIRECTION('center_axis',(0.506912129415013,0.,0.861997733785848));
#20552=DIRECTION('ref_axis',(0.861997733785848,0.,-0.506912129415013));
#20553=DIRECTION('',(-0.861997733785848,0.,0.506912129415013));
#20554=DIRECTION('',(-0.861997733785848,0.,0.506912129415013));
#20555=DIRECTION('center_axis',(0.,1.,0.));
#20556=DIRECTION('ref_axis',(1.,0.,0.));
#20557=DIRECTION('center_axis',(-0.707106781186548,0.,0.707106781186548));
#20558=DIRECTION('ref_axis',(0.707106781186548,0.,0.707106781186548));
#20559=DIRECTION('',(-0.707106781186548,0.,-0.707106781186548));
#20560=DIRECTION('',(0.,1.,0.));
#20561=DIRECTION('',(-0.707106781186548,0.,-0.707106781186548));
#20562=DIRECTION('',(0.,1.,0.));
#20563=DIRECTION('center_axis',(-0.701427359980324,0.,-0.712740947800134));
#20564=DIRECTION('ref_axis',(-0.712740947800134,0.,0.701427359980324));
#20565=DIRECTION('',(0.712740947800134,0.,-0.701427359980324));
#20566=DIRECTION('',(0.712740947800134,0.,-0.701427359980324));
#20567=DIRECTION('',(0.,1.,0.));
#20568=DIRECTION('center_axis',(0.707106781186548,0.,-0.707106781186548));
#20569=DIRECTION('ref_axis',(-0.707106781186548,0.,-0.707106781186548));
#20570=DIRECTION('',(0.707106781186548,0.,0.707106781186548));
#20571=DIRECTION('',(0.707106781186548,0.,0.707106781186548));
#20572=DIRECTION('',(0.,1.,0.));
#20573=DIRECTION('center_axis',(0.712740947800134,0.,0.701427359980324));
#20574=DIRECTION('ref_axis',(0.701427359980324,0.,-0.712740947800134));
#20575=DIRECTION('',(-0.701427359980324,0.,0.712740947800134));
#20576=DIRECTION('',(-0.701427359980324,0.,0.712740947800134));
#20577=DIRECTION('center_axis',(0.,1.,0.));
#20578=DIRECTION('ref_axis',(1.,0.,0.));
#20579=DIRECTION('center_axis',(-0.50000000000003,0.,0.866025403784422));
#20580=DIRECTION('ref_axis',(0.866025403784422,0.,0.50000000000003));
#20581=DIRECTION('',(-0.866025403784422,0.,-0.50000000000003));
#20582=DIRECTION('',(0.,1.,0.));
#20583=DIRECTION('',(-0.866025403784422,0.,-0.50000000000003));
#20584=DIRECTION('',(0.,1.,0.));
#20585=DIRECTION('center_axis',(-0.861997733785848,0.,-0.506912129415013));
#20586=DIRECTION('ref_axis',(-0.506912129415013,0.,0.861997733785848));
#20587=DIRECTION('',(0.506912129415013,0.,-0.861997733785848));
#20588=DIRECTION('',(0.506912129415013,0.,-0.861997733785848));
#20589=DIRECTION('',(0.,1.,0.));
#20590=DIRECTION('center_axis',(0.500000000000001,0.,-0.866025403784438));
#20591=DIRECTION('ref_axis',(-0.866025403784438,0.,-0.500000000000001));
#20592=DIRECTION('',(0.866025403784438,0.,0.500000000000001));
#20593=DIRECTION('',(0.866025403784438,0.,0.500000000000001));
#20594=DIRECTION('',(0.,1.,0.));
#20595=DIRECTION('center_axis',(0.869997648452786,0.,0.49305587075566));
#20596=DIRECTION('ref_axis',(0.49305587075566,0.,-0.869997648452786));
#20597=DIRECTION('',(-0.49305587075566,0.,0.869997648452786));
#20598=DIRECTION('',(-0.49305587075566,0.,0.869997648452786));
#20599=DIRECTION('center_axis',(0.,1.,0.));
#20600=DIRECTION('ref_axis',(1.,0.,0.));
#20601=DIRECTION('center_axis',(-0.258819045102541,0.,0.965925826289063));
#20602=DIRECTION('ref_axis',(0.965925826289063,0.,0.258819045102541));
#20603=DIRECTION('',(-0.965925826289063,0.,-0.258819045102541));
#20604=DIRECTION('',(0.,1.,0.));
#20605=DIRECTION('',(-0.965925826289063,0.,-0.258819045102541));
#20606=DIRECTION('',(0.,1.,0.));
#20607=DIRECTION('center_axis',(-0.963824386552478,0.,-0.26653808712216));
#20608=DIRECTION('ref_axis',(-0.26653808712216,0.,0.963824386552478));
#20609=DIRECTION('',(0.26653808712216,0.,-0.963824386552478));
#20610=DIRECTION('',(0.26653808712216,0.,-0.963824386552478));
#20611=DIRECTION('',(0.,1.,0.));
#20612=DIRECTION('center_axis',(0.258819045102503,0.,-0.965925826289073));
#20613=DIRECTION('ref_axis',(-0.965925826289073,0.,-0.258819045102503));
#20614=DIRECTION('',(0.965925826289073,0.,0.258819045102503));
#20615=DIRECTION('',(0.965925826289073,0.,0.258819045102503));
#20616=DIRECTION('',(0.,1.,0.));
#20617=DIRECTION('center_axis',(0.967965447102477,0.,0.251083438752344));
#20618=DIRECTION('ref_axis',(0.251083438752344,0.,-0.967965447102477));
#20619=DIRECTION('',(-0.251083438752344,0.,0.967965447102477));
#20620=DIRECTION('',(-0.251083438752344,0.,0.967965447102477));
#20621=DIRECTION('center_axis',(0.,1.,0.));
#20622=DIRECTION('ref_axis',(1.,0.,0.));
#20623=DIRECTION('center_axis',(0.,0.,1.));
#20624=DIRECTION('ref_axis',(1.,0.,0.));
#20625=DIRECTION('',(-1.,0.,0.));
#20626=DIRECTION('',(0.,1.,0.));
#20627=DIRECTION('',(-1.,0.,0.));
#20628=DIRECTION('',(0.,1.,0.));
#20629=DIRECTION('center_axis',(-0.999968000170666,0.,-0.00799991466693405));
#20630=DIRECTION('ref_axis',(-0.00799991466693405,0.,0.999968000170666));
#20631=DIRECTION('',(0.00799991466693405,0.,-0.999968000170666));
#20632=DIRECTION('',(0.00799991466693405,0.,-0.999968000170666));
#20633=DIRECTION('',(0.,1.,0.));
#20634=DIRECTION('center_axis',(0.,0.,-1.));
#20635=DIRECTION('ref_axis',(-1.,0.,0.));
#20636=DIRECTION('',(1.,0.,0.));
#20637=DIRECTION('',(1.,0.,0.));
#20638=DIRECTION('',(0.,1.,0.));
#20639=DIRECTION('center_axis',(0.999968000170666,0.,-0.00799991466694293));
#20640=DIRECTION('ref_axis',(-0.00799991466694293,0.,-0.999968000170666));
#20641=DIRECTION('',(0.00799991466694293,0.,0.999968000170666));
#20642=DIRECTION('',(0.00799991466694293,0.,0.999968000170666));
#20643=DIRECTION('center_axis',(0.,1.,0.));
#20644=DIRECTION('ref_axis',(1.,0.,0.));
#20645=DIRECTION('center_axis',(0.258819045102527,0.,0.965925826289067));
#20646=DIRECTION('ref_axis',(0.965925826289067,0.,-0.258819045102527));
#20647=DIRECTION('',(-0.965925826289067,0.,0.258819045102527));
#20648=DIRECTION('',(0.,1.,0.));
#20649=DIRECTION('',(-0.965925826289067,0.,0.258819045102527));
#20650=DIRECTION('',(0.,1.,0.));
#20651=DIRECTION('center_axis',(-0.967965447102479,0.,0.251083438752335));
#20652=DIRECTION('ref_axis',(0.251083438752335,0.,0.967965447102479));
#20653=DIRECTION('',(-0.251083438752335,0.,-0.967965447102479));
#20654=DIRECTION('',(-0.251083438752335,0.,-0.967965447102479));
#20655=DIRECTION('',(0.,1.,0.));
#20656=DIRECTION('center_axis',(-0.258819045102503,0.,-0.965925826289073));
#20657=DIRECTION('ref_axis',(-0.965925826289073,0.,0.258819045102503));
#20658=DIRECTION('',(0.965925826289073,0.,-0.258819045102503));
#20659=DIRECTION('',(0.965925826289073,0.,-0.258819045102503));
#20660=DIRECTION('',(0.,1.,0.));
#20661=DIRECTION('center_axis',(0.963824386552478,0.,-0.26653808712216));
#20662=DIRECTION('ref_axis',(-0.26653808712216,0.,-0.963824386552478));
#20663=DIRECTION('',(0.26653808712216,0.,0.963824386552478));
#20664=DIRECTION('',(0.26653808712216,0.,0.963824386552478));
#20665=DIRECTION('center_axis',(0.,1.,0.));
#20666=DIRECTION('ref_axis',(1.,0.,0.));
#20667=DIRECTION('center_axis',(0.500000000000008,0.,0.866025403784434));
#20668=DIRECTION('ref_axis',(0.866025403784434,0.,-0.500000000000008));
#20669=DIRECTION('',(-0.866025403784434,0.,0.500000000000008));
#20670=DIRECTION('',(0.,1.,0.));
#20671=DIRECTION('',(-0.866025403784434,0.,0.500000000000008));
#20672=DIRECTION('',(0.,1.,0.));
#20673=DIRECTION('center_axis',(-0.86999764845279,0.,0.493055870755653));
#20674=DIRECTION('ref_axis',(0.493055870755653,0.,0.86999764845279));
#20675=DIRECTION('',(-0.493055870755653,0.,-0.86999764845279));
#20676=DIRECTION('',(-0.493055870755653,0.,-0.86999764845279));
#20677=DIRECTION('',(0.,1.,0.));
#20678=DIRECTION('center_axis',(-0.500000000000004,0.,-0.866025403784436));
#20679=DIRECTION('ref_axis',(-0.866025403784436,0.,0.500000000000004));
#20680=DIRECTION('',(0.866025403784436,0.,-0.500000000000004));
#20681=DIRECTION('',(0.866025403784436,0.,-0.500000000000004));
#20682=DIRECTION('',(0.,1.,0.));
#20683=DIRECTION('center_axis',(0.861997733785848,0.,-0.506912129415013));
#20684=DIRECTION('ref_axis',(-0.506912129415013,0.,-0.861997733785848));
#20685=DIRECTION('',(0.506912129415013,0.,0.861997733785848));
#20686=DIRECTION('',(0.506912129415013,0.,0.861997733785848));
#20687=DIRECTION('center_axis',(0.,1.,0.));
#20688=DIRECTION('ref_axis',(1.,0.,0.));
#20689=DIRECTION('center_axis',(0.707106781186533,0.,0.707106781186562));
#20690=DIRECTION('ref_axis',(0.707106781186562,0.,-0.707106781186533));
#20691=DIRECTION('',(-0.707106781186562,0.,0.707106781186533));
#20692=DIRECTION('',(0.,1.,0.));
#20693=DIRECTION('',(-0.707106781186562,0.,0.707106781186533));
#20694=DIRECTION('',(0.,1.,0.));
#20695=DIRECTION('center_axis',(-0.712740947800136,0.,0.701427359980322));
#20696=DIRECTION('ref_axis',(0.701427359980322,0.,0.712740947800136));
#20697=DIRECTION('',(-0.701427359980322,0.,-0.712740947800136));
#20698=DIRECTION('',(-0.701427359980322,0.,-0.712740947800136));
#20699=DIRECTION('',(0.,1.,0.));
#20700=DIRECTION('center_axis',(-0.707106781186564,0.,-0.707106781186531));
#20701=DIRECTION('ref_axis',(-0.707106781186531,0.,0.707106781186564));
#20702=DIRECTION('',(0.707106781186531,0.,-0.707106781186564));
#20703=DIRECTION('',(0.707106781186531,0.,-0.707106781186564));
#20704=DIRECTION('',(0.,1.,0.));
#20705=DIRECTION('center_axis',(0.701427359980322,0.,-0.712740947800136));
#20706=DIRECTION('ref_axis',(-0.712740947800136,0.,-0.701427359980322));
#20707=DIRECTION('',(0.712740947800136,0.,0.701427359980322));
#20708=DIRECTION('',(0.712740947800136,0.,0.701427359980322));
#20709=DIRECTION('center_axis',(0.,1.,0.));
#20710=DIRECTION('ref_axis',(1.,0.,0.));
#20711=DIRECTION('center_axis',(0.866025403784429,0.,0.500000000000017));
#20712=DIRECTION('ref_axis',(0.500000000000017,0.,-0.866025403784429));
#20713=DIRECTION('',(-0.500000000000017,0.,0.866025403784429));
#20714=DIRECTION('',(0.,1.,0.));
#20715=DIRECTION('',(-0.500000000000017,0.,0.866025403784429));
#20716=DIRECTION('',(0.,1.,0.));
#20717=DIRECTION('center_axis',(-0.506912129415013,0.,0.861997733785848));
#20718=DIRECTION('ref_axis',(0.861997733785848,0.,0.506912129415013));
#20719=DIRECTION('',(-0.861997733785848,0.,-0.506912129415013));
#20720=DIRECTION('',(-0.861997733785848,0.,-0.506912129415013));
#20721=DIRECTION('',(0.,1.,0.));
#20722=DIRECTION('center_axis',(-0.866025403784438,0.,-0.500000000000001));
#20723=DIRECTION('ref_axis',(-0.500000000000001,0.,0.866025403784438));
#20724=DIRECTION('',(0.500000000000001,0.,-0.866025403784438));
#20725=DIRECTION('',(0.500000000000001,0.,-0.866025403784438));
#20726=DIRECTION('',(0.,1.,0.));
#20727=DIRECTION('center_axis',(0.493055870755657,0.,-0.869997648452788));
#20728=DIRECTION('ref_axis',(-0.869997648452788,0.,-0.493055870755657));
#20729=DIRECTION('',(0.869997648452788,0.,0.493055870755657));
#20730=DIRECTION('',(0.869997648452788,0.,0.493055870755657));
#20731=DIRECTION('center_axis',(0.,1.,0.));
#20732=DIRECTION('ref_axis',(1.,0.,0.));
#20733=DIRECTION('center_axis',(0.965925826289079,0.,0.258819045102479));
#20734=DIRECTION('ref_axis',(0.258819045102479,0.,-0.965925826289079));
#20735=DIRECTION('',(-0.258819045102479,0.,0.965925826289079));
#20736=DIRECTION('',(0.,1.,0.));
#20737=DIRECTION('',(-0.258819045102479,0.,0.965925826289079));
#20738=DIRECTION('',(0.,1.,0.));
#20739=DIRECTION('center_axis',(-0.266538087122154,0.,0.963824386552479));
#20740=DIRECTION('ref_axis',(0.963824386552479,0.,0.266538087122154));
#20741=DIRECTION('',(-0.963824386552479,0.,-0.266538087122154));
#20742=DIRECTION('',(-0.963824386552479,0.,-0.266538087122154));
#20743=DIRECTION('',(0.,1.,0.));
#20744=DIRECTION('center_axis',(-0.965925826289075,0.,-0.258819045102495));
#20745=DIRECTION('ref_axis',(-0.258819045102495,0.,0.965925826289075));
#20746=DIRECTION('',(0.258819045102495,0.,-0.965925826289075));
#20747=DIRECTION('',(0.258819045102495,0.,-0.965925826289075));
#20748=DIRECTION('',(0.,1.,0.));
#20749=DIRECTION('center_axis',(0.25108343875234,0.,-0.967965447102478));
#20750=DIRECTION('ref_axis',(-0.967965447102478,0.,-0.25108343875234));
#20751=DIRECTION('',(0.967965447102478,0.,0.25108343875234));
#20752=DIRECTION('',(0.967965447102478,0.,0.25108343875234));
#20753=DIRECTION('center_axis',(0.,1.,0.));
#20754=DIRECTION('ref_axis',(1.,0.,0.));
#20755=DIRECTION('center_axis',(1.,0.,0.));
#20756=DIRECTION('ref_axis',(0.,0.,-1.));
#20757=DIRECTION('',(0.,0.,1.));
#20758=DIRECTION('',(0.,1.,0.));
#20759=DIRECTION('',(0.,0.,1.));
#20760=DIRECTION('',(0.,1.,0.));
#20761=DIRECTION('center_axis',(-0.00799991466693849,0.,0.999968000170666));
#20762=DIRECTION('ref_axis',(0.999968000170666,0.,0.00799991466693849));
#20763=DIRECTION('',(-0.999968000170666,0.,-0.00799991466693849));
#20764=DIRECTION('',(-0.999968000170666,0.,-0.00799991466693849));
#20765=DIRECTION('',(0.,1.,0.));
#20766=DIRECTION('center_axis',(-1.,0.,0.));
#20767=DIRECTION('ref_axis',(0.,0.,1.));
#20768=DIRECTION('',(0.,0.,-1.));
#20769=DIRECTION('',(0.,0.,-1.));
#20770=DIRECTION('',(0.,1.,0.));
#20771=DIRECTION('center_axis',(-0.00799991466693849,0.,-0.999968000170666));
#20772=DIRECTION('ref_axis',(-0.999968000170666,0.,0.00799991466693849));
#20773=DIRECTION('',(0.999968000170666,0.,-0.00799991466693849));
#20774=DIRECTION('',(0.999968000170666,0.,-0.00799991466693849));
#20775=DIRECTION('center_axis',(0.,1.,0.));
#20776=DIRECTION('ref_axis',(1.,0.,0.));
#20777=DIRECTION('center_axis',(0.,1.,0.));
#20778=DIRECTION('ref_axis',(1.,0.,0.));
#20779=DIRECTION('center_axis',(0.,1.,0.));
#20780=DIRECTION('ref_axis',(1.,0.,0.));
#20781=DIRECTION('',(0.,1.,0.));
#20782=DIRECTION('center_axis',(0.,-1.,0.));
#20783=DIRECTION('ref_axis',(1.,0.,0.));
#20784=DIRECTION('center_axis',(0.,1.,0.));
#20785=DIRECTION('ref_axis',(1.,0.,0.));
#20786=DIRECTION('center_axis',(0.,1.,0.));
#20787=DIRECTION('ref_axis',(1.,0.,0.));
#20788=DIRECTION('',(0.,1.,0.));
#20789=DIRECTION('center_axis',(0.,-1.,0.));
#20790=DIRECTION('ref_axis',(1.,0.,0.));
#20791=DIRECTION('center_axis',(0.,1.,0.));
#20792=DIRECTION('ref_axis',(1.,0.,0.));
#20793=DIRECTION('center_axis',(0.,1.,0.));
#20794=DIRECTION('ref_axis',(1.,0.,0.));
#20795=DIRECTION('',(0.,1.,0.));
#20796=DIRECTION('center_axis',(0.,-1.,0.));
#20797=DIRECTION('ref_axis',(1.,0.,0.));
#20798=DIRECTION('center_axis',(-1.,0.,0.));
#20799=DIRECTION('ref_axis',(0.,0.,1.));
#20800=DIRECTION('',(0.,1.,0.));
#20801=DIRECTION('',(0.,0.,-1.));
#20802=DIRECTION('',(0.,1.,0.));
#20803=DIRECTION('',(0.,0.,1.));
#20804=DIRECTION('center_axis',(-1.,0.,0.));
#20805=DIRECTION('ref_axis',(0.,0.,1.));
#20806=DIRECTION('',(0.,-1.,0.));
#20807=DIRECTION('',(0.,0.,1.));
#20808=DIRECTION('',(0.,1.,0.));
#20809=DIRECTION('',(0.,0.,-1.));
#20810=DIRECTION('center_axis',(0.,0.,-1.));
#20811=DIRECTION('ref_axis',(-1.,0.,0.));
#20812=DIRECTION('',(1.,0.,0.));
#20813=DIRECTION('',(-1.,0.,0.));
#20814=DIRECTION('',(0.,1.,0.));
#20815=DIRECTION('center_axis',(1.,0.,0.));
#20816=DIRECTION('ref_axis',(0.,0.,-1.));
#20817=DIRECTION('',(0.,0.,1.));
#20818=DIRECTION('',(0.,0.,-1.));
#20819=DIRECTION('',(0.,1.,0.));
#20820=DIRECTION('center_axis',(0.,0.,1.));
#20821=DIRECTION('ref_axis',(1.,0.,0.));
#20822=DIRECTION('',(-1.,0.,0.));
#20823=DIRECTION('',(1.,0.,0.));
#20824=DIRECTION('center_axis',(0.,0.,-1.));
#20825=DIRECTION('ref_axis',(-1.,0.,0.));
#20826=DIRECTION('',(1.,0.,0.));
#20827=DIRECTION('',(0.,-1.,0.));
#20828=DIRECTION('',(-1.,0.,0.));
#20829=DIRECTION('center_axis',(0.,1.,0.));
#20830=DIRECTION('ref_axis',(1.,0.,0.));
#20831=DIRECTION('',(-1.,0.,0.));
#20832=DIRECTION('center_axis',(0.,1.,0.));
#20833=DIRECTION('ref_axis',(1.,0.,0.));
#20834=DIRECTION('center_axis',(0.,0.,1.));
#20835=DIRECTION('ref_axis',(1.,0.,0.));
#20836=DIRECTION('',(1.,0.,0.));
#20837=DIRECTION('',(0.,1.,0.));
#20838=DIRECTION('center_axis',(0.,1.,0.));
#20839=DIRECTION('ref_axis',(1.,0.,0.));
#20840=DIRECTION('center_axis',(0.,1.,0.));
#20841=DIRECTION('ref_axis',(1.,0.,0.));
#20842=DIRECTION('center_axis',(0.,1.,0.));
#20843=DIRECTION('ref_axis',(-1.,0.,-1.22464679914735E-16));
#25157=CARTESIAN_POINT('',(0.,0.,0.));
#25158=CARTESIAN_POINT('Origin',(21.6782686989894,4.15,8.0458829327411));
#25159=CARTESIAN_POINT('',(21.6625326688994,4.2,7.98715526893581));
#25160=CARTESIAN_POINT('',(21.6782686989894,4.2,8.0458829327411));
#25161=CARTESIAN_POINT('',(21.6743346914669,4.2,8.03120101678986));
#25162=CARTESIAN_POINT('',(21.6625326688994,4.15,7.98715526893581));
#25163=CARTESIAN_POINT('',(21.6625326688994,4.15,7.98715526893581));
#25164=CARTESIAN_POINT('',(21.6782686989894,4.15,8.0458829327411));
#25165=CARTESIAN_POINT('',(21.6625326688994,4.15,7.98715526893581));
#25166=CARTESIAN_POINT('',(21.6782686989894,4.15,8.0458829327411));
#25167=CARTESIAN_POINT('Origin',(21.2910825201484,4.15,8.14631630824203));
#25168=CARTESIAN_POINT('',(21.2910825201484,4.2,8.14631630824203));
#25169=CARTESIAN_POINT('',(19.6455412600742,4.2,8.57315815412101));
#25170=CARTESIAN_POINT('',(21.2910825201484,4.15,8.14631630824203));
#25171=CARTESIAN_POINT('',(21.6782686989894,4.15,8.0458829327411));
#25172=CARTESIAN_POINT('',(21.2910825201484,4.15,8.14631630824203));
#25173=CARTESIAN_POINT('Origin',(21.2770029142784,4.15,8.09377050378467));
#25174=CARTESIAN_POINT('',(21.2770029142784,4.2,8.09377050378467));
#25175=CARTESIAN_POINT('',(21.2805228157459,4.2,8.10690695489906));
#25176=CARTESIAN_POINT('',(21.2770029142784,4.15,8.09377050378467));
#25177=CARTESIAN_POINT('',(21.2910825201484,4.15,8.14631630824203));
#25178=CARTESIAN_POINT('',(21.2770029142784,4.15,8.09377050378467));
#25179=CARTESIAN_POINT('Origin',(21.6625326688994,4.15,7.98715526893581));
#25180=CARTESIAN_POINT('',(19.8312663344497,4.2,8.49357763446791));
#25181=CARTESIAN_POINT('',(21.2770029142784,4.15,8.09377050378467));
#25182=CARTESIAN_POINT('Origin',(21.4776358066339,4.15,8.06673578858892));
#25183=CARTESIAN_POINT('Origin',(21.3059910641206,4.15,7.12638769112851));
#25184=CARTESIAN_POINT('',(21.2755913883862,4.2,7.07373390822296));
#25185=CARTESIAN_POINT('',(21.3059910641206,4.2,7.12638769112851));
#25186=CARTESIAN_POINT('',(21.298391145187,4.2,7.11322424540209));
#25187=CARTESIAN_POINT('',(21.2755913883862,4.15,7.07373390822296));
#25188=CARTESIAN_POINT('',(21.2755913883862,4.15,7.07373390822296));
#25189=CARTESIAN_POINT('',(21.3059910641206,4.15,7.12638769112851));
#25190=CARTESIAN_POINT('',(21.2755913883862,4.15,7.07373390822296));
#25191=CARTESIAN_POINT('',(21.3059910641206,4.15,7.12638769112851));
#25192=CARTESIAN_POINT('Origin',(20.9579920047395,4.15,7.32361003943077));
#25193=CARTESIAN_POINT('',(20.9579920047395,4.2,7.32361003943077));
#25194=CARTESIAN_POINT('',(19.4789960023697,4.2,8.16180501971539));
#25195=CARTESIAN_POINT('',(20.9579920047395,4.15,7.32361003943077));
#25196=CARTESIAN_POINT('',(21.3059910641206,4.15,7.12638769112851));
#25197=CARTESIAN_POINT('',(20.9579920047395,4.15,7.32361003943077));
#25198=CARTESIAN_POINT('Origin',(20.9307922948719,4.15,7.27649875998896));
#25199=CARTESIAN_POINT('',(20.9307922948719,4.2,7.27649875998896));
#25200=CARTESIAN_POINT('',(20.9375922223388,4.2,7.28827657984941));
#25201=CARTESIAN_POINT('',(20.9307922948719,4.15,7.27649875998896));
#25202=CARTESIAN_POINT('',(20.9579920047395,4.15,7.32361003943077));
#25203=CARTESIAN_POINT('',(20.9307922948719,4.15,7.27649875998896));
#25204=CARTESIAN_POINT('Origin',(21.2755913883862,4.15,7.07373390822296));
#25205=CARTESIAN_POINT('',(19.6377956941931,4.2,8.03686695411148));
#25206=CARTESIAN_POINT('',(20.9307922948719,4.15,7.27649875998896));
#25207=CARTESIAN_POINT('Origin',(21.1183916794962,4.15,7.19867197382686));
#25208=CARTESIAN_POINT('Origin',(20.7084156016405,4.15,6.33457603207478));
#25209=CARTESIAN_POINT('',(20.6654239679252,4.2,6.29158439835948));
#25210=CARTESIAN_POINT('',(20.7084156016405,4.2,6.33457603207478));
#25211=CARTESIAN_POINT('',(20.6976676932117,4.2,6.32382812364594));
#25212=CARTESIAN_POINT('',(20.6654239679252,4.15,6.29158439835948));
#25213=CARTESIAN_POINT('',(20.6654239679252,4.15,6.29158439835948));
#25214=CARTESIAN_POINT('',(20.7084156016405,4.15,6.33457603207478));
#25215=CARTESIAN_POINT('',(20.6654239679252,4.15,6.29158439835948));
#25216=CARTESIAN_POINT('',(20.7084156016405,4.15,6.33457603207478));
#25217=CARTESIAN_POINT('Origin',(20.4233192225205,4.15,6.6151469760669));
#25218=CARTESIAN_POINT('',(20.4233192225205,4.2,6.6151469760669));
#25219=CARTESIAN_POINT('',(19.2116596112602,4.2,7.80757348803345));
#25220=CARTESIAN_POINT('',(20.4233192225205,4.15,6.6151469760669));
#25221=CARTESIAN_POINT('',(20.7084156016405,4.15,6.33457603207478));
#25222=CARTESIAN_POINT('',(20.4233192225205,4.15,6.6151469760669));
#25223=CARTESIAN_POINT('Origin',(20.3848530239331,4.15,6.57668077747954));
#25224=CARTESIAN_POINT('',(20.3848530239331,4.2,6.57668077747954));
#25225=CARTESIAN_POINT('',(20.39446957358,4.2,6.58629732712641));
#25226=CARTESIAN_POINT('',(20.3848530239331,4.15,6.57668077747954));
#25227=CARTESIAN_POINT('',(20.4233192225205,4.15,6.6151469760669));
#25228=CARTESIAN_POINT('',(20.3848530239331,4.15,6.57668077747954));
#25229=CARTESIAN_POINT('Origin',(20.6654239679252,4.15,6.29158439835948));
#25230=CARTESIAN_POINT('',(19.3327119839626,4.2,7.64579219917974));
#25231=CARTESIAN_POINT('',(20.3848530239331,4.15,6.57668077747954));
#25232=CARTESIAN_POINT('Origin',(20.5466343127868,4.15,6.45336568721319));
#25233=CARTESIAN_POINT('Origin',(19.926266091777,4.15,5.72440861161377));
#25234=CARTESIAN_POINT('',(19.8736123088715,4.2,5.6940089358794));
#25235=CARTESIAN_POINT('',(19.926266091777,4.2,5.72440861161377));
#25236=CARTESIAN_POINT('',(19.9131026460507,4.2,5.71680869268019));
#25237=CARTESIAN_POINT('',(19.8736123088715,4.15,5.6940089358794));
#25238=CARTESIAN_POINT('',(19.8736123088715,4.15,5.6940089358794));
#25239=CARTESIAN_POINT('',(19.926266091777,4.15,5.72440861161377));
#25240=CARTESIAN_POINT('',(19.8736123088715,4.15,5.6940089358794));
#25241=CARTESIAN_POINT('',(19.926266091777,4.15,5.72440861161377));
#25242=CARTESIAN_POINT('Origin',(19.723501240011,4.15,6.06920770512811));
#25243=CARTESIAN_POINT('',(19.723501240011,4.2,6.06920770512811));
#25244=CARTESIAN_POINT('',(18.8617506200055,4.2,7.53460385256405));
#25245=CARTESIAN_POINT('',(19.723501240011,4.15,6.06920770512811));
#25246=CARTESIAN_POINT('',(19.926266091777,4.15,5.72440861161377));
#25247=CARTESIAN_POINT('',(19.723501240011,4.15,6.06920770512811));
#25248=CARTESIAN_POINT('Origin',(19.6763899605692,4.15,6.04200799526052));
#25249=CARTESIAN_POINT('',(19.6763899605692,4.2,6.04200799526052));
#25250=CARTESIAN_POINT('',(19.6881677804297,4.2,6.04880792272743));
#25251=CARTESIAN_POINT('',(19.6763899605692,4.15,6.04200799526052));
#25252=CARTESIAN_POINT('',(19.723501240011,4.15,6.06920770512811));
#25253=CARTESIAN_POINT('',(19.6763899605692,4.15,6.04200799526052));
#25254=CARTESIAN_POINT('Origin',(19.8736123088715,4.15,5.6940089358794));
#25255=CARTESIAN_POINT('',(18.9368061544358,4.2,7.3470044679397));
#25256=CARTESIAN_POINT('',(19.6763899605692,4.15,6.04200799526052));
#25257=CARTESIAN_POINT('Origin',(19.8013280261731,4.15,5.88160832050376));
#25258=CARTESIAN_POINT('Origin',(19.0128447310642,4.15,5.33746733110058));
#25259=CARTESIAN_POINT('',(18.9541170672589,4.2,5.32173130101059));
#25260=CARTESIAN_POINT('',(19.0128447310642,4.2,5.33746733110058));
#25261=CARTESIAN_POINT('',(18.9981628151129,4.2,5.33353332357809));
#25262=CARTESIAN_POINT('',(18.9541170672589,4.15,5.32173130101059));
#25263=CARTESIAN_POINT('',(18.9541170672589,4.15,5.32173130101059));
#25264=CARTESIAN_POINT('',(19.0128447310642,4.15,5.33746733110058));
#25265=CARTESIAN_POINT('',(18.9541170672589,4.15,5.32173130101059));
#25266=CARTESIAN_POINT('',(19.0128447310642,4.15,5.33746733110058));
#25267=CARTESIAN_POINT('Origin',(18.9062294962153,4.15,5.72299708572157));
#25268=CARTESIAN_POINT('',(18.9062294962153,4.2,5.72299708572157));
#25269=CARTESIAN_POINT('',(18.4531147481077,4.2,7.36149854286079));
#25270=CARTESIAN_POINT('',(18.9062294962153,4.15,5.72299708572157));
#25271=CARTESIAN_POINT('',(19.0128447310642,4.15,5.33746733110058));
#25272=CARTESIAN_POINT('',(18.9062294962153,4.15,5.72299708572157));
#25273=CARTESIAN_POINT('Origin',(18.853683691758,4.15,5.70891747985158));
#25274=CARTESIAN_POINT('',(18.853683691758,4.2,5.70891747985158));
#25275=CARTESIAN_POINT('',(18.8668201428723,4.2,5.71243738131908));
#25276=CARTESIAN_POINT('',(18.853683691758,4.15,5.70891747985158));
#25277=CARTESIAN_POINT('',(18.9062294962153,4.15,5.72299708572157));
#25278=CARTESIAN_POINT('',(18.853683691758,4.15,5.70891747985158));
#25279=CARTESIAN_POINT('Origin',(18.9541170672589,4.15,5.32173130101059));
#25280=CARTESIAN_POINT('',(18.4770585336294,4.2,7.16086565050529));
#25281=CARTESIAN_POINT('',(18.853683691758,4.15,5.70891747985158));
#25282=CARTESIAN_POINT('Origin',(18.9332642114111,4.15,5.52236419336608));
#25283=CARTESIAN_POINT('Origin',(18.0303996757344,4.15,5.20012159935147));
#25284=CARTESIAN_POINT('',(17.9696003242656,4.2,5.20012159935147));
#25285=CARTESIAN_POINT('',(18.0303996757344,4.2,5.20012159935147));
#25286=CARTESIAN_POINT('',(18.0151998378672,4.2,5.20012159935147));
#25287=CARTESIAN_POINT('',(17.9696003242656,4.15,5.20012159935147));
#25288=CARTESIAN_POINT('',(17.9696003242656,4.15,5.20012159935147));
#25289=CARTESIAN_POINT('',(18.0303996757344,4.15,5.20012159935147));
#25290=CARTESIAN_POINT('',(17.9696003242656,4.15,5.20012159935147));
#25291=CARTESIAN_POINT('',(18.0303996757344,4.15,5.20012159935147));
#25292=CARTESIAN_POINT('Origin',(18.0271997098676,4.15,5.60010879941973));
#25293=CARTESIAN_POINT('',(18.0271997098676,4.2,5.60010879941973));
#25294=CARTESIAN_POINT('',(18.0135998549338,4.2,7.30005439970987));
#25295=CARTESIAN_POINT('',(18.0271997098676,4.15,5.60010879941973));
#25296=CARTESIAN_POINT('',(18.0303996757344,4.15,5.20012159935147));
#25297=CARTESIAN_POINT('',(18.0271997098676,4.15,5.60010879941973));
#25298=CARTESIAN_POINT('Origin',(17.9728002901324,4.15,5.60010879941973));
#25299=CARTESIAN_POINT('',(17.9728002901324,4.2,5.60010879941973));
#25300=CARTESIAN_POINT('',(17.9864001450662,4.2,5.60010879941973));
#25301=CARTESIAN_POINT('',(17.9728002901324,4.15,5.60010879941973));
#25302=CARTESIAN_POINT('',(18.0271997098676,4.15,5.60010879941973));
#25303=CARTESIAN_POINT('',(17.9728002901324,4.15,5.60010879941973));
#25304=CARTESIAN_POINT('Origin',(17.9696003242656,4.15,5.20012159935147));
#25305=CARTESIAN_POINT('',(17.9848001621328,4.2,7.10006079967573));
#25306=CARTESIAN_POINT('',(17.9728002901324,4.15,5.60010879941973));
#25307=CARTESIAN_POINT('Origin',(18.,4.15,5.4001151993856));
#25308=CARTESIAN_POINT('Origin',(17.0458829327411,4.15,5.32173130101059));
#25309=CARTESIAN_POINT('',(16.9871552689358,4.2,5.33746733110058));
#25310=CARTESIAN_POINT('',(17.0458829327411,4.2,5.32173130101059));
#25311=CARTESIAN_POINT('',(17.0312010167898,4.2,5.32566530853307));
#25312=CARTESIAN_POINT('',(16.9871552689358,4.15,5.33746733110058));
#25313=CARTESIAN_POINT('',(16.9871552689358,4.15,5.33746733110058));
#25314=CARTESIAN_POINT('',(17.0458829327411,4.15,5.32173130101059));
#25315=CARTESIAN_POINT('',(16.9871552689358,4.15,5.33746733110058));
#25316=CARTESIAN_POINT('',(17.0458829327411,4.15,5.32173130101059));
#25317=CARTESIAN_POINT('Origin',(17.146316308242,4.15,5.70891747985158));
#25318=CARTESIAN_POINT('',(17.146316308242,4.2,5.70891747985158));
#25319=CARTESIAN_POINT('',(17.573158154121,4.2,7.35445873992579));
#25320=CARTESIAN_POINT('',(17.146316308242,4.15,5.70891747985158));
#25321=CARTESIAN_POINT('',(17.0458829327411,4.15,5.32173130101059));
#25322=CARTESIAN_POINT('',(17.146316308242,4.15,5.70891747985158));
#25323=CARTESIAN_POINT('Origin',(17.0937705037847,4.15,5.72299708572157));
#25324=CARTESIAN_POINT('',(17.0937705037847,4.2,5.72299708572157));
#25325=CARTESIAN_POINT('',(17.106906954899,4.2,5.71947718425408));
#25326=CARTESIAN_POINT('',(17.0937705037847,4.15,5.72299708572157));
#25327=CARTESIAN_POINT('',(17.146316308242,4.15,5.70891747985158));
#25328=CARTESIAN_POINT('',(17.0937705037847,4.15,5.72299708572157));
#25329=CARTESIAN_POINT('Origin',(16.9871552689358,4.15,5.33746733110058));
#25330=CARTESIAN_POINT('',(17.4935776344679,4.2,7.16873366555029));
#25331=CARTESIAN_POINT('',(17.0937705037847,4.15,5.72299708572157));
#25332=CARTESIAN_POINT('Origin',(17.0667357885889,4.15,5.52236419336608));
#25333=CARTESIAN_POINT('Origin',(16.1263876911285,4.15,5.6940089358794));
#25334=CARTESIAN_POINT('',(16.073733908223,4.2,5.72440861161377));
#25335=CARTESIAN_POINT('',(16.1263876911285,4.2,5.6940089358794));
#25336=CARTESIAN_POINT('',(16.1132242454022,4.2,5.70160885481298));
#25337=CARTESIAN_POINT('',(16.073733908223,4.15,5.72440861161377));
#25338=CARTESIAN_POINT('',(16.073733908223,4.15,5.72440861161377));
#25339=CARTESIAN_POINT('',(16.1263876911285,4.15,5.6940089358794));
#25340=CARTESIAN_POINT('',(16.073733908223,4.15,5.72440861161377));
#25341=CARTESIAN_POINT('',(16.1263876911285,4.15,5.6940089358794));
#25342=CARTESIAN_POINT('Origin',(16.3236100394308,4.15,6.04200799526052));
#25343=CARTESIAN_POINT('',(16.3236100394308,4.2,6.04200799526052));
#25344=CARTESIAN_POINT('',(17.1618050197154,4.2,7.52100399763026));
#25345=CARTESIAN_POINT('',(16.3236100394308,4.15,6.04200799526052));
#25346=CARTESIAN_POINT('',(16.1263876911285,4.15,5.6940089358794));
#25347=CARTESIAN_POINT('',(16.3236100394308,4.15,6.04200799526052));
#25348=CARTESIAN_POINT('Origin',(16.276498759989,4.15,6.06920770512811));
#25349=CARTESIAN_POINT('',(16.276498759989,4.2,6.06920770512811));
#25350=CARTESIAN_POINT('',(16.2882765798494,4.2,6.06240777766122));
#25351=CARTESIAN_POINT('',(16.276498759989,4.15,6.06920770512811));
#25352=CARTESIAN_POINT('',(16.3236100394308,4.15,6.04200799526052));
#25353=CARTESIAN_POINT('',(16.276498759989,4.15,6.06920770512811));
#25354=CARTESIAN_POINT('Origin',(16.073733908223,4.15,5.72440861161377));
#25355=CARTESIAN_POINT('',(17.0368669541115,4.2,7.36220430580689));
#25356=CARTESIAN_POINT('',(16.276498759989,4.15,6.06920770512811));
#25357=CARTESIAN_POINT('Origin',(16.1986719738269,4.15,5.88160832050376));
#25358=CARTESIAN_POINT('Origin',(15.3345760320748,4.15,6.29158439835949));
#25359=CARTESIAN_POINT('',(15.2915843983595,4.2,6.33457603207478));
#25360=CARTESIAN_POINT('',(15.3345760320748,4.2,6.29158439835949));
#25361=CARTESIAN_POINT('',(15.3238281236459,4.2,6.30233230678832));
#25362=CARTESIAN_POINT('',(15.2915843983595,4.15,6.33457603207478));
#25363=CARTESIAN_POINT('',(15.2915843983595,4.15,6.33457603207478));
#25364=CARTESIAN_POINT('',(15.3345760320748,4.15,6.29158439835949));
#25365=CARTESIAN_POINT('',(15.2915843983595,4.15,6.33457603207478));
#25366=CARTESIAN_POINT('',(15.3345760320748,4.15,6.29158439835949));
#25367=CARTESIAN_POINT('Origin',(15.6151469760669,4.15,6.57668077747954));
#25368=CARTESIAN_POINT('',(15.6151469760669,4.2,6.57668077747954));
#25369=CARTESIAN_POINT('',(16.8075734880335,4.2,7.78834038873977));
#25370=CARTESIAN_POINT('',(15.6151469760669,4.15,6.57668077747954));
#25371=CARTESIAN_POINT('',(15.3345760320748,4.15,6.29158439835949));
#25372=CARTESIAN_POINT('',(15.6151469760669,4.15,6.57668077747954));
#25373=CARTESIAN_POINT('Origin',(15.5766807774795,4.15,6.61514697606691));
#25374=CARTESIAN_POINT('',(15.5766807774795,4.2,6.61514697606691));
#25375=CARTESIAN_POINT('',(15.5862973271264,4.2,6.60553042642005));
#25376=CARTESIAN_POINT('',(15.5766807774795,4.15,6.61514697606691));
#25377=CARTESIAN_POINT('',(15.6151469760669,4.15,6.57668077747954));
#25378=CARTESIAN_POINT('',(15.5766807774795,4.15,6.61514697606691));
#25379=CARTESIAN_POINT('Origin',(15.2915843983595,4.15,6.33457603207478));
#25380=CARTESIAN_POINT('',(16.6457921991797,4.2,7.66728801603739));
#25381=CARTESIAN_POINT('',(15.5766807774795,4.15,6.61514697606691));
#25382=CARTESIAN_POINT('Origin',(15.4533656872132,4.15,6.4533656872132));
#25383=CARTESIAN_POINT('Origin',(14.7244086116138,4.15,7.07373390822296));
#25384=CARTESIAN_POINT('',(14.6940089358794,4.2,7.12638769112851));
#25385=CARTESIAN_POINT('',(14.7244086116138,4.2,7.07373390822296));
#25386=CARTESIAN_POINT('',(14.7168086926802,4.2,7.0868973539493));
#25387=CARTESIAN_POINT('',(14.6940089358794,4.15,7.12638769112851));
#25388=CARTESIAN_POINT('',(14.6940089358794,4.15,7.12638769112851));
#25389=CARTESIAN_POINT('',(14.7244086116138,4.15,7.07373390822296));
#25390=CARTESIAN_POINT('',(14.6940089358794,4.15,7.12638769112851));
#25391=CARTESIAN_POINT('',(14.7244086116138,4.15,7.07373390822296));
#25392=CARTESIAN_POINT('Origin',(15.0692077051281,4.15,7.27649875998896));
#25393=CARTESIAN_POINT('',(15.0692077051281,4.2,7.27649875998896));
#25394=CARTESIAN_POINT('',(16.5346038525641,4.2,8.13824937999448));
#25395=CARTESIAN_POINT('',(15.0692077051281,4.15,7.27649875998896));
#25396=CARTESIAN_POINT('',(14.7244086116138,4.15,7.07373390822296));
#25397=CARTESIAN_POINT('',(15.0692077051281,4.15,7.27649875998896));
#25398=CARTESIAN_POINT('Origin',(15.0420079952605,4.15,7.32361003943077));
#25399=CARTESIAN_POINT('',(15.0420079952605,4.2,7.32361003943077));
#25400=CARTESIAN_POINT('',(15.0488079227274,4.2,7.31183221957035));
#25401=CARTESIAN_POINT('',(15.0420079952605,4.15,7.32361003943077));
#25402=CARTESIAN_POINT('',(15.0692077051281,4.15,7.27649875998896));
#25403=CARTESIAN_POINT('',(15.0420079952605,4.15,7.32361003943077));
#25404=CARTESIAN_POINT('Origin',(14.6940089358794,4.15,7.12638769112851));
#25405=CARTESIAN_POINT('',(16.3470044679397,4.2,8.06319384556425));
#25406=CARTESIAN_POINT('',(15.0420079952605,4.15,7.32361003943077));
#25407=CARTESIAN_POINT('Origin',(14.8816083205038,4.15,7.19867197382687));
#25408=CARTESIAN_POINT('Origin',(14.3374673311006,4.15,7.98715526893581));
#25409=CARTESIAN_POINT('',(14.3217313010106,4.2,8.0458829327411));
#25410=CARTESIAN_POINT('',(14.3374673311006,4.2,7.98715526893581));
#25411=CARTESIAN_POINT('',(14.3335333235781,4.2,8.00183718488717));
#25412=CARTESIAN_POINT('',(14.3217313010106,4.15,8.0458829327411));
#25413=CARTESIAN_POINT('',(14.3217313010106,4.15,8.0458829327411));
#25414=CARTESIAN_POINT('',(14.3374673311006,4.15,7.98715526893581));
#25415=CARTESIAN_POINT('',(14.3217313010106,4.15,8.0458829327411));
#25416=CARTESIAN_POINT('',(14.3374673311006,4.15,7.98715526893581));
#25417=CARTESIAN_POINT('Origin',(14.7229970857216,4.15,8.09377050378467));
#25418=CARTESIAN_POINT('',(14.7229970857216,4.2,8.09377050378467));
#25419=CARTESIAN_POINT('',(16.3614985428608,4.2,8.54688525189233));
#25420=CARTESIAN_POINT('',(14.7229970857216,4.15,8.09377050378467));
#25421=CARTESIAN_POINT('',(14.3374673311006,4.15,7.98715526893581));
#25422=CARTESIAN_POINT('',(14.7229970857216,4.15,8.09377050378467));
#25423=CARTESIAN_POINT('Origin',(14.7089174798516,4.15,8.14631630824203));
#25424=CARTESIAN_POINT('',(14.7089174798516,4.2,8.14631630824203));
#25425=CARTESIAN_POINT('',(14.7124373813191,4.2,8.13317985712775));
#25426=CARTESIAN_POINT('',(14.7089174798516,4.15,8.14631630824203));
#25427=CARTESIAN_POINT('',(14.7229970857216,4.15,8.09377050378467));
#25428=CARTESIAN_POINT('',(14.7089174798516,4.15,8.14631630824203));
#25429=CARTESIAN_POINT('Origin',(14.3217313010106,4.15,8.0458829327411));
#25430=CARTESIAN_POINT('',(16.1608656505053,4.2,8.52294146637054));
#25431=CARTESIAN_POINT('',(14.7089174798516,4.15,8.14631630824203));
#25432=CARTESIAN_POINT('Origin',(14.5223641933661,4.15,8.06673578858892));
#25433=CARTESIAN_POINT('Origin',(14.2001215993515,4.15,8.96960032426563));
#25434=CARTESIAN_POINT('',(14.2001215993515,4.2,9.03039967573437));
#25435=CARTESIAN_POINT('',(14.2001215993515,4.2,8.96960032426563));
#25436=CARTESIAN_POINT('',(14.2001215993515,4.2,8.98480016213281));
#25437=CARTESIAN_POINT('',(14.2001215993515,4.15,9.03039967573437));
#25438=CARTESIAN_POINT('',(14.2001215993515,4.15,9.03039967573437));
#25439=CARTESIAN_POINT('',(14.2001215993515,4.15,8.96960032426563));
#25440=CARTESIAN_POINT('',(14.2001215993515,4.15,9.03039967573437));
#25441=CARTESIAN_POINT('',(14.2001215993515,4.15,8.96960032426563));
#25442=CARTESIAN_POINT('Origin',(14.6001087994197,4.15,8.9728002901324));
#25443=CARTESIAN_POINT('',(14.6001087994197,4.2,8.9728002901324));
#25444=CARTESIAN_POINT('',(16.3000543997099,4.2,8.9864001450662));
#25445=CARTESIAN_POINT('',(14.6001087994197,4.15,8.9728002901324));
#25446=CARTESIAN_POINT('',(14.2001215993515,4.15,8.96960032426563));
#25447=CARTESIAN_POINT('',(14.6001087994197,4.15,8.9728002901324));
#25448=CARTESIAN_POINT('Origin',(14.6001087994197,4.15,9.0271997098676));
#25449=CARTESIAN_POINT('',(14.6001087994197,4.2,9.0271997098676));
#25450=CARTESIAN_POINT('',(14.6001087994197,4.2,9.0135998549338));
#25451=CARTESIAN_POINT('',(14.6001087994197,4.15,9.0271997098676));
#25452=CARTESIAN_POINT('',(14.6001087994197,4.15,8.9728002901324));
#25453=CARTESIAN_POINT('',(14.6001087994197,4.15,9.0271997098676));
#25454=CARTESIAN_POINT('Origin',(14.2001215993515,4.15,9.03039967573437));
#25455=CARTESIAN_POINT('',(16.1000607996757,4.2,9.01519983786719));
#25456=CARTESIAN_POINT('',(14.6001087994197,4.15,9.0271997098676));
#25457=CARTESIAN_POINT('Origin',(14.4001151993856,4.15,9.));
#25458=CARTESIAN_POINT('Origin',(14.3217313010106,4.15,9.95411706725891));
#25459=CARTESIAN_POINT('',(14.3374673311006,4.2,10.0128447310642));
#25460=CARTESIAN_POINT('',(14.3217313010106,4.2,9.95411706725891));
#25461=CARTESIAN_POINT('',(14.3256653085331,4.2,9.96879898321025));
#25462=CARTESIAN_POINT('',(14.3374673311006,4.15,10.0128447310642));
#25463=CARTESIAN_POINT('',(14.3374673311006,4.15,10.0128447310642));
#25464=CARTESIAN_POINT('',(14.3217313010106,4.15,9.95411706725891));
#25465=CARTESIAN_POINT('',(14.3374673311006,4.15,10.0128447310642));
#25466=CARTESIAN_POINT('',(14.3217313010106,4.15,9.95411706725891));
#25467=CARTESIAN_POINT('Origin',(14.7089174798516,4.15,9.85368369175797));
#25468=CARTESIAN_POINT('',(14.7089174798516,4.2,9.85368369175797));
#25469=CARTESIAN_POINT('',(16.3544587399258,4.2,9.42684184587898));
#25470=CARTESIAN_POINT('',(14.7089174798516,4.15,9.85368369175797));
#25471=CARTESIAN_POINT('',(14.3217313010106,4.15,9.95411706725891));
#25472=CARTESIAN_POINT('',(14.7089174798516,4.15,9.85368369175797));
#25473=CARTESIAN_POINT('Origin',(14.7229970857216,4.15,9.90622949621533));
#25474=CARTESIAN_POINT('',(14.7229970857216,4.2,9.90622949621533));
#25475=CARTESIAN_POINT('',(14.7194771842541,4.2,9.89309304510103));
#25476=CARTESIAN_POINT('',(14.7229970857216,4.15,9.90622949621533));
#25477=CARTESIAN_POINT('',(14.7089174798516,4.15,9.85368369175797));
#25478=CARTESIAN_POINT('',(14.7229970857216,4.15,9.90622949621533));
#25479=CARTESIAN_POINT('Origin',(14.3374673311006,4.15,10.0128447310642));
#25480=CARTESIAN_POINT('',(16.1687336655503,4.2,9.5064223655321));
#25481=CARTESIAN_POINT('',(14.7229970857216,4.15,9.90622949621533));
#25482=CARTESIAN_POINT('Origin',(14.5223641933661,4.15,9.93326421141108));
#25483=CARTESIAN_POINT('Origin',(14.6940089358794,4.15,10.8736123088715));
#25484=CARTESIAN_POINT('',(14.7244086116138,4.2,10.926266091777));
#25485=CARTESIAN_POINT('',(14.6940089358794,4.2,10.8736123088715));
#25486=CARTESIAN_POINT('',(14.701608854813,4.2,10.8867757545979));
#25487=CARTESIAN_POINT('',(14.7244086116138,4.15,10.926266091777));
#25488=CARTESIAN_POINT('',(14.7244086116138,4.15,10.926266091777));
#25489=CARTESIAN_POINT('',(14.6940089358794,4.15,10.8736123088715));
#25490=CARTESIAN_POINT('',(14.7244086116138,4.15,10.926266091777));
#25491=CARTESIAN_POINT('',(14.6940089358794,4.15,10.8736123088715));
#25492=CARTESIAN_POINT('Origin',(15.0420079952605,4.15,10.6763899605692));
#25493=CARTESIAN_POINT('',(15.0420079952605,4.2,10.6763899605692));
#25494=CARTESIAN_POINT('',(16.5210039976303,4.2,9.83819498028462));
#25495=CARTESIAN_POINT('',(15.0420079952605,4.15,10.6763899605692));
#25496=CARTESIAN_POINT('',(14.6940089358794,4.15,10.8736123088715));
#25497=CARTESIAN_POINT('',(15.0420079952605,4.15,10.6763899605692));
#25498=CARTESIAN_POINT('Origin',(15.0692077051281,4.15,10.723501240011));
#25499=CARTESIAN_POINT('',(15.0692077051281,4.2,10.723501240011));
#25500=CARTESIAN_POINT('',(15.0624077776612,4.2,10.7117234201505));
#25501=CARTESIAN_POINT('',(15.0692077051281,4.15,10.723501240011));
#25502=CARTESIAN_POINT('',(15.0420079952605,4.15,10.6763899605692));
#25503=CARTESIAN_POINT('',(15.0692077051281,4.15,10.723501240011));
#25504=CARTESIAN_POINT('Origin',(14.7244086116138,4.15,10.926266091777));
#25505=CARTESIAN_POINT('',(16.3622043058069,4.2,9.96313304588852));
#25506=CARTESIAN_POINT('',(15.0692077051281,4.15,10.723501240011));
#25507=CARTESIAN_POINT('Origin',(14.8816083205038,4.15,10.8013280261731));
#25508=CARTESIAN_POINT('Origin',(15.2915843983595,4.15,11.6654239679252));
#25509=CARTESIAN_POINT('',(15.3345760320748,4.2,11.7084156016405));
#25510=CARTESIAN_POINT('',(15.2915843983595,4.2,11.6654239679252));
#25511=CARTESIAN_POINT('',(15.3023323067883,4.2,11.676171876354));
#25512=CARTESIAN_POINT('',(15.3345760320748,4.15,11.7084156016405));
#25513=CARTESIAN_POINT('',(15.3345760320748,4.15,11.7084156016405));
#25514=CARTESIAN_POINT('',(15.2915843983595,4.15,11.6654239679252));
#25515=CARTESIAN_POINT('',(15.3345760320748,4.15,11.7084156016405));
#25516=CARTESIAN_POINT('',(15.2915843983595,4.15,11.6654239679252));
#25517=CARTESIAN_POINT('Origin',(15.5766807774795,4.15,11.3848530239331));
#25518=CARTESIAN_POINT('',(15.5766807774795,4.2,11.3848530239331));
#25519=CARTESIAN_POINT('',(16.7883403887398,4.2,10.1924265119665));
#25520=CARTESIAN_POINT('',(15.5766807774795,4.15,11.3848530239331));
#25521=CARTESIAN_POINT('',(15.2915843983595,4.15,11.6654239679252));
#25522=CARTESIAN_POINT('',(15.5766807774795,4.15,11.3848530239331));
#25523=CARTESIAN_POINT('Origin',(15.6151469760669,4.15,11.4233192225205));
#25524=CARTESIAN_POINT('',(15.6151469760669,4.2,11.4233192225205));
#25525=CARTESIAN_POINT('',(15.6055304264201,4.2,11.4137026728736));
#25526=CARTESIAN_POINT('',(15.6151469760669,4.15,11.4233192225205));
#25527=CARTESIAN_POINT('',(15.5766807774795,4.15,11.3848530239331));
#25528=CARTESIAN_POINT('',(15.6151469760669,4.15,11.4233192225205));
#25529=CARTESIAN_POINT('Origin',(15.3345760320748,4.15,11.7084156016405));
#25530=CARTESIAN_POINT('',(16.6672880160374,4.2,10.3542078008203));
#25531=CARTESIAN_POINT('',(15.6151469760669,4.15,11.4233192225205));
#25532=CARTESIAN_POINT('Origin',(15.4533656872132,4.15,11.5466343127868));
#25533=CARTESIAN_POINT('Origin',(16.073733908223,4.15,12.2755913883862));
#25534=CARTESIAN_POINT('',(16.1263876911285,4.2,12.3059910641206));
#25535=CARTESIAN_POINT('',(16.073733908223,4.2,12.2755913883862));
#25536=CARTESIAN_POINT('',(16.0868973539493,4.2,12.2831913073198));
#25537=CARTESIAN_POINT('',(16.1263876911285,4.15,12.3059910641206));
#25538=CARTESIAN_POINT('',(16.1263876911285,4.15,12.3059910641206));
#25539=CARTESIAN_POINT('',(16.073733908223,4.15,12.2755913883862));
#25540=CARTESIAN_POINT('',(16.1263876911285,4.15,12.3059910641206));
#25541=CARTESIAN_POINT('',(16.073733908223,4.15,12.2755913883862));
#25542=CARTESIAN_POINT('Origin',(16.276498759989,4.15,11.9307922948719));
#25543=CARTESIAN_POINT('',(16.276498759989,4.2,11.9307922948719));
#25544=CARTESIAN_POINT('',(17.1382493799945,4.2,10.4653961474359));
#25545=CARTESIAN_POINT('',(16.276498759989,4.15,11.9307922948719));
#25546=CARTESIAN_POINT('',(16.073733908223,4.15,12.2755913883862));
#25547=CARTESIAN_POINT('',(16.276498759989,4.15,11.9307922948719));
#25548=CARTESIAN_POINT('Origin',(16.3236100394308,4.15,11.9579920047395));
#25549=CARTESIAN_POINT('',(16.3236100394308,4.2,11.9579920047395));
#25550=CARTESIAN_POINT('',(16.3118322195703,4.2,11.9511920772726));
#25551=CARTESIAN_POINT('',(16.3236100394308,4.15,11.9579920047395));
#25552=CARTESIAN_POINT('',(16.276498759989,4.15,11.9307922948719));
#25553=CARTESIAN_POINT('',(16.3236100394308,4.15,11.9579920047395));
#25554=CARTESIAN_POINT('Origin',(16.1263876911285,4.15,12.3059910641206));
#25555=CARTESIAN_POINT('',(17.0631938455643,4.2,10.6529955320603));
#25556=CARTESIAN_POINT('',(16.3236100394308,4.15,11.9579920047395));
#25557=CARTESIAN_POINT('Origin',(16.1986719738269,4.15,12.1183916794962));
#25558=CARTESIAN_POINT('Origin',(16.9871552689358,4.15,12.6625326688994));
#25559=CARTESIAN_POINT('',(17.0458829327411,4.2,12.6782686989894));
#25560=CARTESIAN_POINT('',(16.9871552689358,4.2,12.6625326688994));
#25561=CARTESIAN_POINT('',(17.0018371848871,4.2,12.6664666764219));
#25562=CARTESIAN_POINT('',(17.0458829327411,4.15,12.6782686989894));
#25563=CARTESIAN_POINT('',(17.0458829327411,4.15,12.6782686989894));
#25564=CARTESIAN_POINT('',(16.9871552689358,4.15,12.6625326688994));
#25565=CARTESIAN_POINT('',(17.0458829327411,4.15,12.6782686989894));
#25566=CARTESIAN_POINT('',(16.9871552689358,4.15,12.6625326688994));
#25567=CARTESIAN_POINT('Origin',(17.0937705037847,4.15,12.2770029142784));
#25568=CARTESIAN_POINT('',(17.0937705037847,4.2,12.2770029142784));
#25569=CARTESIAN_POINT('',(17.5468852518923,4.2,10.6385014571392));
#25570=CARTESIAN_POINT('',(17.0937705037847,4.15,12.2770029142784));
#25571=CARTESIAN_POINT('',(16.9871552689358,4.15,12.6625326688994));
#25572=CARTESIAN_POINT('',(17.0937705037847,4.15,12.2770029142784));
#25573=CARTESIAN_POINT('Origin',(17.146316308242,4.15,12.2910825201484));
#25574=CARTESIAN_POINT('',(17.146316308242,4.2,12.2910825201484));
#25575=CARTESIAN_POINT('',(17.1331798571277,4.2,12.2875626186809));
#25576=CARTESIAN_POINT('',(17.146316308242,4.15,12.2910825201484));
#25577=CARTESIAN_POINT('',(17.0937705037847,4.15,12.2770029142784));
#25578=CARTESIAN_POINT('',(17.146316308242,4.15,12.2910825201484));
#25579=CARTESIAN_POINT('Origin',(17.0458829327411,4.15,12.6782686989894));
#25580=CARTESIAN_POINT('',(17.5229414663705,4.2,10.8391343494947));
#25581=CARTESIAN_POINT('',(17.146316308242,4.15,12.2910825201484));
#25582=CARTESIAN_POINT('Origin',(17.0667357885889,4.15,12.4776358066339));
#25583=CARTESIAN_POINT('Origin',(17.9696003242656,4.15,12.7998784006485));
#25584=CARTESIAN_POINT('',(18.0303996757344,4.2,12.7998784006485));
#25585=CARTESIAN_POINT('',(17.9696003242656,4.2,12.7998784006485));
#25586=CARTESIAN_POINT('',(17.9848001621328,4.2,12.7998784006485));
#25587=CARTESIAN_POINT('',(18.0303996757344,4.15,12.7998784006485));
#25588=CARTESIAN_POINT('',(18.0303996757344,4.15,12.7998784006485));
#25589=CARTESIAN_POINT('',(17.9696003242656,4.15,12.7998784006485));
#25590=CARTESIAN_POINT('',(18.0303996757344,4.15,12.7998784006485));
#25591=CARTESIAN_POINT('',(17.9696003242656,4.15,12.7998784006485));
#25592=CARTESIAN_POINT('Origin',(17.9728002901324,4.15,12.3998912005803));
#25593=CARTESIAN_POINT('',(17.9728002901324,4.2,12.3998912005803));
#25594=CARTESIAN_POINT('',(17.9864001450662,4.2,10.6999456002901));
#25595=CARTESIAN_POINT('',(17.9728002901324,4.15,12.3998912005803));
#25596=CARTESIAN_POINT('',(17.9696003242656,4.15,12.7998784006485));
#25597=CARTESIAN_POINT('',(17.9728002901324,4.15,12.3998912005803));
#25598=CARTESIAN_POINT('Origin',(18.0271997098676,4.15,12.3998912005803));
#25599=CARTESIAN_POINT('',(18.0271997098676,4.2,12.3998912005803));
#25600=CARTESIAN_POINT('',(18.0135998549338,4.2,12.3998912005803));
#25601=CARTESIAN_POINT('',(18.0271997098676,4.15,12.3998912005803));
#25602=CARTESIAN_POINT('',(17.9728002901324,4.15,12.3998912005803));
#25603=CARTESIAN_POINT('',(18.0271997098676,4.15,12.3998912005803));
#25604=CARTESIAN_POINT('Origin',(18.0303996757344,4.15,12.7998784006485));
#25605=CARTESIAN_POINT('',(18.0151998378672,4.2,10.8999392003243));
#25606=CARTESIAN_POINT('',(18.0271997098676,4.15,12.3998912005803));
#25607=CARTESIAN_POINT('Origin',(18.,4.15,12.5998848006144));
#25608=CARTESIAN_POINT('Origin',(18.9541170672589,4.15,12.6782686989894));
#25609=CARTESIAN_POINT('',(19.0128447310642,4.2,12.6625326688994));
#25610=CARTESIAN_POINT('',(18.9541170672589,4.2,12.6782686989894));
#25611=CARTESIAN_POINT('',(18.9687989832102,4.2,12.6743346914669));
#25612=CARTESIAN_POINT('',(19.0128447310642,4.15,12.6625326688994));
#25613=CARTESIAN_POINT('',(19.0128447310642,4.15,12.6625326688994));
#25614=CARTESIAN_POINT('',(18.9541170672589,4.15,12.6782686989894));
#25615=CARTESIAN_POINT('',(19.0128447310642,4.15,12.6625326688994));
#25616=CARTESIAN_POINT('',(18.9541170672589,4.15,12.6782686989894));
#25617=CARTESIAN_POINT('Origin',(18.853683691758,4.15,12.2910825201484));
#25618=CARTESIAN_POINT('',(18.853683691758,4.2,12.2910825201484));
#25619=CARTESIAN_POINT('',(18.426841845879,4.2,10.6455412600742));
#25620=CARTESIAN_POINT('',(18.853683691758,4.15,12.2910825201484));
#25621=CARTESIAN_POINT('',(18.9541170672589,4.15,12.6782686989894));
#25622=CARTESIAN_POINT('',(18.853683691758,4.15,12.2910825201484));
#25623=CARTESIAN_POINT('Origin',(18.9062294962153,4.15,12.2770029142784));
#25624=CARTESIAN_POINT('',(18.9062294962153,4.2,12.2770029142784));
#25625=CARTESIAN_POINT('',(18.893093045101,4.2,12.2805228157459));
#25626=CARTESIAN_POINT('',(18.9062294962153,4.15,12.2770029142784));
#25627=CARTESIAN_POINT('',(18.853683691758,4.15,12.2910825201484));
#25628=CARTESIAN_POINT('',(18.9062294962153,4.15,12.2770029142784));
#25629=CARTESIAN_POINT('Origin',(19.0128447310642,4.15,12.6625326688994));
#25630=CARTESIAN_POINT('',(18.5064223655321,4.2,10.8312663344497));
#25631=CARTESIAN_POINT('',(18.9062294962153,4.15,12.2770029142784));
#25632=CARTESIAN_POINT('Origin',(18.9332642114111,4.15,12.4776358066339));
#25633=CARTESIAN_POINT('Origin',(19.8736123088715,4.15,12.3059910641206));
#25634=CARTESIAN_POINT('',(19.926266091777,4.2,12.2755913883862));
#25635=CARTESIAN_POINT('',(19.8736123088715,4.2,12.3059910641206));
#25636=CARTESIAN_POINT('',(19.8867757545979,4.2,12.298391145187));
#25637=CARTESIAN_POINT('',(19.926266091777,4.15,12.2755913883862));
#25638=CARTESIAN_POINT('',(19.926266091777,4.15,12.2755913883862));
#25639=CARTESIAN_POINT('',(19.8736123088715,4.15,12.3059910641206));
#25640=CARTESIAN_POINT('',(19.926266091777,4.15,12.2755913883862));
#25641=CARTESIAN_POINT('',(19.8736123088715,4.15,12.3059910641206));
#25642=CARTESIAN_POINT('Origin',(19.6763899605692,4.15,11.9579920047395));
#25643=CARTESIAN_POINT('',(19.6763899605692,4.2,11.9579920047395));
#25644=CARTESIAN_POINT('',(18.8381949802846,4.2,10.4789960023697));
#25645=CARTESIAN_POINT('',(19.6763899605692,4.15,11.9579920047395));
#25646=CARTESIAN_POINT('',(19.8736123088715,4.15,12.3059910641206));
#25647=CARTESIAN_POINT('',(19.6763899605692,4.15,11.9579920047395));
#25648=CARTESIAN_POINT('Origin',(19.723501240011,4.15,11.9307922948719));
#25649=CARTESIAN_POINT('',(19.723501240011,4.2,11.9307922948719));
#25650=CARTESIAN_POINT('',(19.7117234201506,4.2,11.9375922223388));
#25651=CARTESIAN_POINT('',(19.723501240011,4.15,11.9307922948719));
#25652=CARTESIAN_POINT('',(19.6763899605692,4.15,11.9579920047395));
#25653=CARTESIAN_POINT('',(19.723501240011,4.15,11.9307922948719));
#25654=CARTESIAN_POINT('Origin',(19.926266091777,4.15,12.2755913883862));
#25655=CARTESIAN_POINT('',(18.9631330458885,4.2,10.6377956941931));
#25656=CARTESIAN_POINT('',(19.723501240011,4.15,11.9307922948719));
#25657=CARTESIAN_POINT('Origin',(19.8013280261731,4.15,12.1183916794962));
#25658=CARTESIAN_POINT('Origin',(20.6654239679252,4.15,11.7084156016405));
#25659=CARTESIAN_POINT('',(20.7084156016405,4.2,11.6654239679252));
#25660=CARTESIAN_POINT('',(20.6654239679252,4.2,11.7084156016405));
#25661=CARTESIAN_POINT('',(20.676171876354,4.2,11.6976676932117));
#25662=CARTESIAN_POINT('',(20.7084156016405,4.15,11.6654239679252));
#25663=CARTESIAN_POINT('',(20.7084156016405,4.15,11.6654239679252));
#25664=CARTESIAN_POINT('',(20.6654239679252,4.15,11.7084156016405));
#25665=CARTESIAN_POINT('',(20.7084156016405,4.15,11.6654239679252));
#25666=CARTESIAN_POINT('',(20.6654239679252,4.15,11.7084156016405));
#25667=CARTESIAN_POINT('Origin',(20.3848530239331,4.15,11.4233192225205));
#25668=CARTESIAN_POINT('',(20.3848530239331,4.2,11.4233192225205));
#25669=CARTESIAN_POINT('',(19.1924265119665,4.2,10.2116596112602));
#25670=CARTESIAN_POINT('',(20.3848530239331,4.15,11.4233192225205));
#25671=CARTESIAN_POINT('',(20.6654239679252,4.15,11.7084156016405));
#25672=CARTESIAN_POINT('',(20.3848530239331,4.15,11.4233192225205));
#25673=CARTESIAN_POINT('Origin',(20.4233192225205,4.15,11.3848530239331));
#25674=CARTESIAN_POINT('',(20.4233192225205,4.2,11.3848530239331));
#25675=CARTESIAN_POINT('',(20.4137026728736,4.2,11.3944695735799));
#25676=CARTESIAN_POINT('',(20.4233192225205,4.15,11.3848530239331));
#25677=CARTESIAN_POINT('',(20.3848530239331,4.15,11.4233192225205));
#25678=CARTESIAN_POINT('',(20.4233192225205,4.15,11.3848530239331));
#25679=CARTESIAN_POINT('Origin',(20.7084156016405,4.15,11.6654239679252));
#25680=CARTESIAN_POINT('',(19.3542078008203,4.2,10.3327119839626));
#25681=CARTESIAN_POINT('',(20.4233192225205,4.15,11.3848530239331));
#25682=CARTESIAN_POINT('Origin',(20.5466343127868,4.15,11.5466343127868));
#25683=CARTESIAN_POINT('Origin',(21.2755913883862,4.15,10.926266091777));
#25684=CARTESIAN_POINT('',(21.3059910641206,4.2,10.8736123088715));
#25685=CARTESIAN_POINT('',(21.2755913883862,4.2,10.926266091777));
#25686=CARTESIAN_POINT('',(21.2831913073198,4.2,10.9131026460507));
#25687=CARTESIAN_POINT('',(21.3059910641206,4.15,10.8736123088715));
#25688=CARTESIAN_POINT('',(21.3059910641206,4.15,10.8736123088715));
#25689=CARTESIAN_POINT('',(21.2755913883862,4.15,10.926266091777));
#25690=CARTESIAN_POINT('',(21.3059910641206,4.15,10.8736123088715));
#25691=CARTESIAN_POINT('',(21.2755913883862,4.15,10.926266091777));
#25692=CARTESIAN_POINT('Origin',(20.9307922948719,4.15,10.723501240011));
#25693=CARTESIAN_POINT('',(20.9307922948719,4.2,10.723501240011));
#25694=CARTESIAN_POINT('',(19.4653961474359,4.2,9.86175062000551));
#25695=CARTESIAN_POINT('',(20.9307922948719,4.15,10.723501240011));
#25696=CARTESIAN_POINT('',(21.2755913883862,4.15,10.926266091777));
#25697=CARTESIAN_POINT('',(20.9307922948719,4.15,10.723501240011));
#25698=CARTESIAN_POINT('Origin',(20.9579920047395,4.15,10.6763899605692));
#25699=CARTESIAN_POINT('',(20.9579920047395,4.2,10.6763899605692));
#25700=CARTESIAN_POINT('',(20.9511920772726,4.2,10.6881677804297));
#25701=CARTESIAN_POINT('',(20.9579920047395,4.15,10.6763899605692));
#25702=CARTESIAN_POINT('',(20.9307922948719,4.15,10.723501240011));
#25703=CARTESIAN_POINT('',(20.9579920047395,4.15,10.6763899605692));
#25704=CARTESIAN_POINT('Origin',(21.3059910641206,4.15,10.8736123088715));
#25705=CARTESIAN_POINT('',(19.6529955320603,4.2,9.93680615443574));
#25706=CARTESIAN_POINT('',(20.9579920047395,4.15,10.6763899605692));
#25707=CARTESIAN_POINT('Origin',(21.1183916794962,4.15,10.8013280261731));
#25708=CARTESIAN_POINT('Origin',(21.6625326688994,4.15,10.0128447310642));
#25709=CARTESIAN_POINT('',(21.6782686989894,4.2,9.9541170672589));
#25710=CARTESIAN_POINT('',(21.6625326688994,4.2,10.0128447310642));
#25711=CARTESIAN_POINT('',(21.6664666764219,4.2,9.99816281511279));
#25712=CARTESIAN_POINT('',(21.6782686989894,4.15,9.9541170672589));
#25713=CARTESIAN_POINT('',(21.6782686989894,4.15,9.9541170672589));
#25714=CARTESIAN_POINT('',(21.6625326688994,4.15,10.0128447310642));
#25715=CARTESIAN_POINT('',(21.6782686989894,4.15,9.9541170672589));
#25716=CARTESIAN_POINT('',(21.6625326688994,4.15,10.0128447310642));
#25717=CARTESIAN_POINT('Origin',(21.2770029142784,4.15,9.90622949621533));
#25718=CARTESIAN_POINT('',(21.2770029142784,4.2,9.90622949621533));
#25719=CARTESIAN_POINT('',(19.6385014571392,4.2,9.45311474810766));
#25720=CARTESIAN_POINT('',(21.2770029142784,4.15,9.90622949621533));
#25721=CARTESIAN_POINT('',(21.6625326688994,4.15,10.0128447310642));
#25722=CARTESIAN_POINT('',(21.2770029142784,4.15,9.90622949621533));
#25723=CARTESIAN_POINT('Origin',(21.2910825201484,4.15,9.85368369175797));
#25724=CARTESIAN_POINT('',(21.2910825201484,4.2,9.85368369175797));
#25725=CARTESIAN_POINT('',(21.2875626186809,4.2,9.86682014287226));
#25726=CARTESIAN_POINT('',(21.2910825201484,4.15,9.85368369175797));
#25727=CARTESIAN_POINT('',(21.2770029142784,4.15,9.90622949621533));
#25728=CARTESIAN_POINT('',(21.2910825201484,4.15,9.85368369175797));
#25729=CARTESIAN_POINT('Origin',(21.6782686989894,4.15,9.9541170672589));
#25730=CARTESIAN_POINT('',(19.8391343494947,4.2,9.47705853362946));
#25731=CARTESIAN_POINT('',(21.2910825201484,4.15,9.85368369175797));
#25732=CARTESIAN_POINT('Origin',(21.4776358066339,4.15,9.93326421141108));
#25733=CARTESIAN_POINT('Origin',(21.7998784006485,4.15,9.03039967573437));
#25734=CARTESIAN_POINT('',(21.7998784006485,4.2,8.96960032426563));
#25735=CARTESIAN_POINT('',(21.7998784006485,4.2,9.03039967573437));
#25736=CARTESIAN_POINT('',(21.7998784006485,4.2,9.01519983786719));
#25737=CARTESIAN_POINT('',(21.7998784006485,4.15,8.96960032426563));
#25738=CARTESIAN_POINT('',(21.7998784006485,4.15,8.96960032426563));
#25739=CARTESIAN_POINT('',(21.7998784006485,4.15,9.03039967573437));
#25740=CARTESIAN_POINT('',(21.7998784006485,4.15,8.96960032426563));
#25741=CARTESIAN_POINT('',(21.7998784006485,4.15,9.03039967573437));
#25742=CARTESIAN_POINT('Origin',(21.3998912005803,4.15,9.0271997098676));
#25743=CARTESIAN_POINT('',(21.3998912005803,4.2,9.0271997098676));
#25744=CARTESIAN_POINT('',(19.6999456002901,4.2,9.0135998549338));
#25745=CARTESIAN_POINT('',(21.3998912005803,4.15,9.0271997098676));
#25746=CARTESIAN_POINT('',(21.7998784006485,4.15,9.03039967573437));
#25747=CARTESIAN_POINT('',(21.3998912005803,4.15,9.0271997098676));
#25748=CARTESIAN_POINT('Origin',(21.3998912005803,4.15,8.9728002901324));
#25749=CARTESIAN_POINT('',(21.3998912005803,4.2,8.9728002901324));
#25750=CARTESIAN_POINT('',(21.3998912005803,4.2,8.9864001450662));
#25751=CARTESIAN_POINT('',(21.3998912005803,4.15,8.9728002901324));
#25752=CARTESIAN_POINT('',(21.3998912005803,4.15,9.0271997098676));
#25753=CARTESIAN_POINT('',(21.3998912005803,4.15,8.9728002901324));
#25754=CARTESIAN_POINT('Origin',(21.7998784006485,4.15,8.96960032426563));
#25755=CARTESIAN_POINT('',(19.8999392003243,4.2,8.98480016213281));
#25756=CARTESIAN_POINT('',(21.3998912005803,4.15,8.9728002901324));
#25757=CARTESIAN_POINT('Origin',(21.5998848006144,4.15,9.));
#25758=CARTESIAN_POINT('Origin',(23.,3.7,14.));
#25759=CARTESIAN_POINT('',(22.775,3.8,14.));
#25760=CARTESIAN_POINT('Origin',(23.,3.8,14.));
#25761=CARTESIAN_POINT('',(22.775,4.2,14.));
#25762=CARTESIAN_POINT('',(22.775,3.7,14.));
#25763=CARTESIAN_POINT('Origin',(23.,4.2,14.));
#25764=CARTESIAN_POINT('Origin',(23.,3.7,4.));
#25765=CARTESIAN_POINT('',(22.775,3.8,4.));
#25766=CARTESIAN_POINT('Origin',(23.,3.8,4.));
#25767=CARTESIAN_POINT('',(22.775,4.2,4.));
#25768=CARTESIAN_POINT('',(22.775,3.7,4.));
#25769=CARTESIAN_POINT('Origin',(23.,4.2,4.));
#25770=CARTESIAN_POINT('Origin',(18.,3.7,9.));
#25771=CARTESIAN_POINT('',(16.475,3.8,9.));
#25772=CARTESIAN_POINT('Origin',(18.,3.8,9.));
#25773=CARTESIAN_POINT('',(16.475,4.2,9.));
#25774=CARTESIAN_POINT('',(16.475,3.7,9.));
#25775=CARTESIAN_POINT('Origin',(18.,4.2,9.));
#25776=CARTESIAN_POINT('Origin',(22.5,3.8,3.5));
#25777=CARTESIAN_POINT('',(22.5,3.8,9.5));
#25778=CARTESIAN_POINT('',(22.5,4.2,9.5));
#25779=CARTESIAN_POINT('',(22.5,3.8,9.5));
#25780=CARTESIAN_POINT('',(22.5,3.8,14.5));
#25781=CARTESIAN_POINT('',(22.5,3.8,14.5));
#25782=CARTESIAN_POINT('',(22.5,4.2,14.5));
#25783=CARTESIAN_POINT('',(22.5,3.8,14.5));
#25784=CARTESIAN_POINT('',(22.5,4.2,14.5));
#25785=CARTESIAN_POINT('Origin',(22.5,3.8,3.5));
#25786=CARTESIAN_POINT('',(22.5,4.2,8.5));
#25787=CARTESIAN_POINT('',(22.5,3.8,8.5));
#25788=CARTESIAN_POINT('',(22.5,3.8,8.5));
#25789=CARTESIAN_POINT('',(22.5,4.2,3.5));
#25790=CARTESIAN_POINT('',(22.5,4.2,14.5));
#25791=CARTESIAN_POINT('',(22.5,3.8,3.5));
#25792=CARTESIAN_POINT('',(22.5,3.8,3.5));
#25793=CARTESIAN_POINT('',(22.5,3.8,14.5));
#25794=CARTESIAN_POINT('Origin',(23.5,3.8,3.5));
#25795=CARTESIAN_POINT('',(23.5,3.8,3.5));
#25796=CARTESIAN_POINT('',(22.5,3.8,3.5));
#25797=CARTESIAN_POINT('',(23.5,4.2,3.5));
#25798=CARTESIAN_POINT('',(22.5,4.2,3.5));
#25799=CARTESIAN_POINT('',(23.5,3.8,3.5));
#25800=CARTESIAN_POINT('Origin',(23.5,3.8,14.5));
#25801=CARTESIAN_POINT('',(23.5,3.8,14.5));
#25802=CARTESIAN_POINT('',(23.5,3.8,3.5));
#25803=CARTESIAN_POINT('',(23.5,4.2,14.5));
#25804=CARTESIAN_POINT('',(23.5,4.2,3.5));
#25805=CARTESIAN_POINT('',(23.5,3.8,14.5));
#25806=CARTESIAN_POINT('Origin',(22.5,3.8,14.5));
#25807=CARTESIAN_POINT('',(23.5,3.8,14.5));
#25808=CARTESIAN_POINT('',(23.5,4.2,14.5));
#25809=CARTESIAN_POINT('Origin',(23.,3.8,8.5));
#25810=CARTESIAN_POINT('',(21.9686269665969,3.8,8.5));
#25811=CARTESIAN_POINT('',(18.,3.8,8.5));
#25812=CARTESIAN_POINT('',(21.9686269665969,4.2,8.5));
#25813=CARTESIAN_POINT('',(21.9686269665969,3.8,8.5));
#25814=CARTESIAN_POINT('',(18.,4.2,8.5));
#25815=CARTESIAN_POINT('Origin',(18.,3.8,9.));
#25816=CARTESIAN_POINT('',(21.9686269665969,3.8,9.5));
#25817=CARTESIAN_POINT('',(23.,3.8,9.5));
#25818=CARTESIAN_POINT('Origin',(18.,3.8,9.));
#25819=CARTESIAN_POINT('Origin',(18.,3.8,9.5));
#25820=CARTESIAN_POINT('',(21.9686269665969,4.2,9.5));
#25821=CARTESIAN_POINT('',(23.,4.2,9.5));
#25822=CARTESIAN_POINT('',(21.9686269665969,3.8,9.5));
#25823=CARTESIAN_POINT('Origin',(18.,4.2,9.));
#25824=CARTESIAN_POINT('Origin',(18.,4.2,9.));
#25825=CARTESIAN_POINT('Origin',(18.,3.8,9.));
#62637=UNCERTAINTY_MEASURE_WITH_UNIT(LENGTH_MEASURE(0.001),#62759,
'DISTANCE_ACCURACY_VALUE',
'Maximum model space distance between geometric entities at asserted c
onnectivities');
#62684=UNCERTAINTY_MEASURE_WITH_UNIT(LENGTH_MEASURE(0.001),#62759,
'DISTANCE_ACCURACY_VALUE',
'Maximum model space distance between geometric entities at asserted c
onnectivities');
#62711=(
GEOMETRIC_REPRESENTATION_CONTEXT(3)
GLOBAL_UNCERTAINTY_ASSIGNED_CONTEXT((#62637))
GLOBAL_UNIT_ASSIGNED_CONTEXT((#62759,#62761,#62762))
REPRESENTATION_CONTEXT('','3D')
);
#62758=(
GEOMETRIC_REPRESENTATION_CONTEXT(3)
GLOBAL_UNCERTAINTY_ASSIGNED_CONTEXT((#62684))
GLOBAL_UNIT_ASSIGNED_CONTEXT((#62759,#62761,#62762))
REPRESENTATION_CONTEXT('','3D')
);
#62759=(
LENGTH_UNIT()
NAMED_UNIT(*)
SI_UNIT(.CENTI.,.METRE.)
);
#62761=(
NAMED_UNIT(*)
PLANE_ANGLE_UNIT()
SI_UNIT($,.RADIAN.)
);
#62762=(
NAMED_UNIT(*)
SI_UNIT($,.STERADIAN.)
SOLID_ANGLE_UNIT()
);
#62789=SHAPE_DEFINITION_REPRESENTATION(#62872,#63057);
#62872=PRODUCT_DEFINITION_SHAPE('',$,#63131);
#63057=SHAPE_REPRESENTATION('',(#17770),#62711);
#63104=PRODUCT_DEFINITION_CONTEXT('part definition',#63325,'design');
#63131=PRODUCT_DEFINITION('Output dial','Output dial',#63204,#63104);
#63204=PRODUCT_DEFINITION_FORMATION('',$,#63353);
#63325=APPLICATION_CONTEXT(
'Core Data for Automotive Mechanical Design Process');
#63326=PRODUCT_CONTEXT('part definition',#63325,'mechanical');
#63353=PRODUCT('Output dial','Output dial','Output dial',(#63326));
#63470=COLOUR_RGB('Off White',0.89,0.88,0.83);
#63471=FILL_AREA_STYLE_COLOUR('',#63470);
#63472=FILL_AREA_STYLE('',(#63471));
#63473=SURFACE_STYLE_FILL_AREA(#63472);
#63474=SURFACE_SIDE_STYLE('',(#63473));
#63475=SURFACE_STYLE_USAGE(.BOTH.,#63474);
#63476=PRESENTATION_STYLE_ASSIGNMENT((#63475));
ENDSEC;
END-ISO-10303-21;
